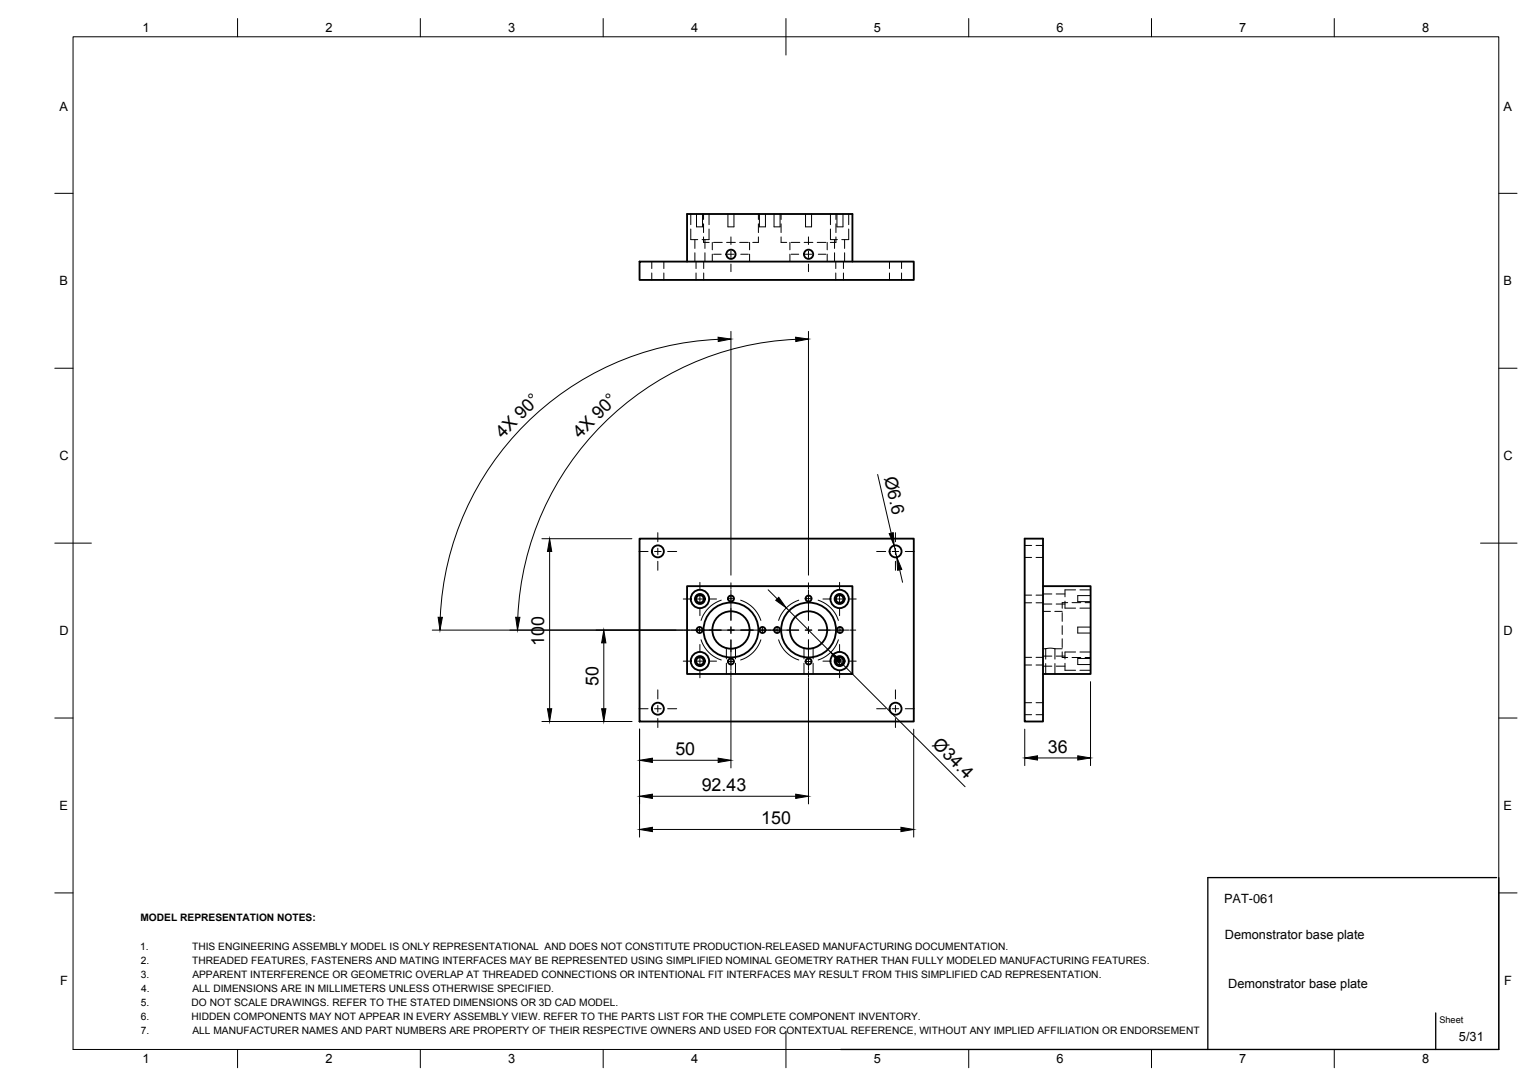
ISO-10303-21;
HEADER;
/* Generated by software containing ST-Developer
 * from STEP Tools, Inc. (www.steptools.com) 
 */

FILE_DESCRIPTION(
/* description */ ('Compact intermittent indexer'),
/* implementation_level */ '2;1');

FILE_NAME(
/* name */ 'Demonstrator base plate.step',
/* time_stamp */ '2026-10-29T16:32:17-07:00',
/* author */ (''),
/* organization */ (''),
/* preprocessor_version */ 'ST-DEVELOPER v20.2',
/* originating_system */ 'Autodesk Translation Framework v15.17.0.0',
/* authorisation */ '');

FILE_SCHEMA (('AUTOMOTIVE_DESIGN { 1 0 10303 214 3 1 1 }'));
ENDSEC;

DATA;
#10=MECHANICAL_DESIGN_GEOMETRIC_PRESENTATION_REPRESENTATION('',(#257),#10837);
#209=SHAPE_REPRESENTATION_RELATIONSHIP('SRR','None',#10943,#233);
#233=ADVANCED_BREP_SHAPE_REPRESENTATION('',(#289),#10810);
#257=STYLED_ITEM('',(#11145),#289);
#289=MANIFOLD_SOLID_BREP('Body1',#5629);
#319=B_SPLINE_CURVE_WITH_KNOTS('',3,(#8545,#8546,#8547,#8548,#8549,#8550,
#8551,#8552,#8553,#8554,#8555,#8556,#8557,#8558,#8559,#8560,#8561,#8562,
#8563,#8564,#8565,#8566,#8567,#8568,#8569,#8570,#8571,#8572,#8573,#8574,
#8575,#8576,#8577,#8578),.UNSPECIFIED.,.T.,.F.,(4,2,2,2,2,2,2,2,2,2,2,2,
2,2,2,2,4),(0.,0.094594182476448,0.189188364952896,0.283770357603024,0.378352350253152,
0.472934342903279,0.567516335553407,0.662110518029855,0.756704700506303,
0.851298882982751,0.945893065459199,1.04047505810933,1.13505705075945,1.22963904340958,
1.32422103605971,1.41881521853616,1.51340940101261),.UNSPECIFIED.);
#320=B_SPLINE_CURVE_WITH_KNOTS('',3,(#8621,#8622,#8623,#8624,#8625,#8626,
#8627,#8628,#8629,#8630,#8631,#8632,#8633,#8634,#8635,#8636,#8637,#8638,
#8639,#8640,#8641,#8642,#8643,#8644,#8645,#8646,#8647,#8648,#8649,#8650,
#8651,#8652,#8653,#8654),.UNSPECIFIED.,.T.,.F.,(4,2,2,2,2,2,2,2,2,2,2,2,
2,2,2,2,4),(0.,0.0945941824764479,0.189188364952896,0.283770357603024,0.378352350253152,
0.47293434290328,0.567516335553408,0.662110518029856,0.756704700506303,
0.851298882982751,0.945893065459199,1.04047505810933,1.13505705075946,1.22963904340958,
1.32422103605971,1.41881521853616,1.51340940101261),.UNSPECIFIED.);
#359=FACE_BOUND('',#996,.T.);
#360=FACE_BOUND('',#998,.T.);
#361=FACE_BOUND('',#1009,.T.);
#362=FACE_BOUND('',#1011,.T.);
#363=FACE_BOUND('',#1014,.T.);
#364=FACE_BOUND('',#1017,.T.);
#365=FACE_BOUND('',#1020,.T.);
#366=FACE_BOUND('',#1023,.T.);
#367=FACE_BOUND('',#1029,.T.);
#368=FACE_BOUND('',#1031,.T.);
#369=FACE_BOUND('',#1033,.T.);
#370=FACE_BOUND('',#1035,.T.);
#371=FACE_BOUND('',#1044,.T.);
#372=FACE_BOUND('',#1045,.T.);
#373=FACE_BOUND('',#1046,.T.);
#374=FACE_BOUND('',#1047,.T.);
#375=FACE_BOUND('',#1048,.T.);
#376=FACE_BOUND('',#1049,.T.);
#377=FACE_BOUND('',#1050,.T.);
#378=FACE_BOUND('',#1051,.T.);
#379=FACE_BOUND('',#1052,.T.);
#380=FACE_BOUND('',#1053,.T.);
#381=FACE_BOUND('',#1054,.T.);
#382=FACE_BOUND('',#1055,.T.);
#383=FACE_BOUND('',#1056,.T.);
#384=FACE_BOUND('',#1057,.T.);
#385=FACE_BOUND('',#1059,.T.);
#386=FACE_BOUND('',#1060,.T.);
#387=FACE_BOUND('',#1074,.T.);
#388=FACE_BOUND('',#1075,.T.);
#389=FACE_BOUND('',#1076,.T.);
#390=FACE_BOUND('',#1077,.T.);
#391=FACE_BOUND('',#1078,.T.);
#392=FACE_BOUND('',#1080,.T.);
#393=FACE_BOUND('',#1081,.T.);
#394=FACE_BOUND('',#1082,.T.);
#395=FACE_BOUND('',#1083,.T.);
#396=FACE_BOUND('',#1084,.T.);
#397=FACE_BOUND('',#1085,.T.);
#398=FACE_BOUND('',#1086,.T.);
#399=FACE_BOUND('',#1087,.T.);
#471=PLANE('',#5934);
#472=PLANE('',#5938);
#473=PLANE('',#5942);
#474=PLANE('',#5946);
#475=PLANE('',#5950);
#476=PLANE('',#5957);
#477=PLANE('',#5961);
#478=PLANE('',#5965);
#479=PLANE('',#5969);
#480=PLANE('',#5973);
#481=PLANE('',#5980);
#482=PLANE('',#5985);
#483=PLANE('',#5990);
#484=PLANE('',#5995);
#485=PLANE('',#6005);
#486=PLANE('',#6007);
#487=PLANE('',#6009);
#488=PLANE('',#6011);
#489=PLANE('',#6013);
#490=PLANE('',#6014);
#491=PLANE('',#6015);
#492=PLANE('',#6016);
#493=PLANE('',#6017);
#494=PLANE('',#6022);
#495=PLANE('',#6023);
#496=PLANE('',#6036);
#497=PLANE('',#6037);
#498=PLANE('',#6038);
#499=PLANE('',#6039);
#500=PLANE('',#6048);
#501=PLANE('',#6049);
#652=FACE_OUTER_BOUND('',#986,.T.);
#653=FACE_OUTER_BOUND('',#987,.T.);
#654=FACE_OUTER_BOUND('',#988,.T.);
#655=FACE_OUTER_BOUND('',#989,.T.);
#656=FACE_OUTER_BOUND('',#990,.T.);
#657=FACE_OUTER_BOUND('',#991,.T.);
#658=FACE_OUTER_BOUND('',#992,.T.);
#659=FACE_OUTER_BOUND('',#993,.T.);
#660=FACE_OUTER_BOUND('',#994,.T.);
#661=FACE_OUTER_BOUND('',#995,.T.);
#662=FACE_OUTER_BOUND('',#997,.T.);
#663=FACE_OUTER_BOUND('',#999,.T.);
#664=FACE_OUTER_BOUND('',#1000,.T.);
#665=FACE_OUTER_BOUND('',#1001,.T.);
#666=FACE_OUTER_BOUND('',#1002,.T.);
#667=FACE_OUTER_BOUND('',#1003,.T.);
#668=FACE_OUTER_BOUND('',#1004,.T.);
#669=FACE_OUTER_BOUND('',#1005,.T.);
#670=FACE_OUTER_BOUND('',#1006,.T.);
#671=FACE_OUTER_BOUND('',#1007,.T.);
#672=FACE_OUTER_BOUND('',#1008,.T.);
#673=FACE_OUTER_BOUND('',#1010,.T.);
#674=FACE_OUTER_BOUND('',#1012,.T.);
#675=FACE_OUTER_BOUND('',#1013,.T.);
#676=FACE_OUTER_BOUND('',#1015,.T.);
#677=FACE_OUTER_BOUND('',#1016,.T.);
#678=FACE_OUTER_BOUND('',#1018,.T.);
#679=FACE_OUTER_BOUND('',#1019,.T.);
#680=FACE_OUTER_BOUND('',#1021,.T.);
#681=FACE_OUTER_BOUND('',#1022,.T.);
#682=FACE_OUTER_BOUND('',#1024,.T.);
#683=FACE_OUTER_BOUND('',#1025,.T.);
#684=FACE_OUTER_BOUND('',#1026,.T.);
#685=FACE_OUTER_BOUND('',#1027,.T.);
#686=FACE_OUTER_BOUND('',#1028,.T.);
#687=FACE_OUTER_BOUND('',#1030,.T.);
#688=FACE_OUTER_BOUND('',#1032,.T.);
#689=FACE_OUTER_BOUND('',#1034,.T.);
#690=FACE_OUTER_BOUND('',#1036,.T.);
#691=FACE_OUTER_BOUND('',#1037,.T.);
#692=FACE_OUTER_BOUND('',#1038,.T.);
#693=FACE_OUTER_BOUND('',#1039,.T.);
#694=FACE_OUTER_BOUND('',#1040,.T.);
#695=FACE_OUTER_BOUND('',#1041,.T.);
#696=FACE_OUTER_BOUND('',#1042,.T.);
#697=FACE_OUTER_BOUND('',#1043,.T.);
#698=FACE_OUTER_BOUND('',#1058,.T.);
#699=FACE_OUTER_BOUND('',#1061,.T.);
#700=FACE_OUTER_BOUND('',#1062,.T.);
#701=FACE_OUTER_BOUND('',#1063,.T.);
#702=FACE_OUTER_BOUND('',#1064,.T.);
#703=FACE_OUTER_BOUND('',#1065,.T.);
#704=FACE_OUTER_BOUND('',#1066,.T.);
#705=FACE_OUTER_BOUND('',#1067,.T.);
#706=FACE_OUTER_BOUND('',#1068,.T.);
#707=FACE_OUTER_BOUND('',#1069,.T.);
#708=FACE_OUTER_BOUND('',#1070,.T.);
#709=FACE_OUTER_BOUND('',#1071,.T.);
#710=FACE_OUTER_BOUND('',#1072,.T.);
#711=FACE_OUTER_BOUND('',#1073,.T.);
#712=FACE_OUTER_BOUND('',#1079,.T.);
#986=EDGE_LOOP('',(#3708,#3709,#3710,#3711));
#987=EDGE_LOOP('',(#3712));
#988=EDGE_LOOP('',(#3713,#3714,#3715,#3716));
#989=EDGE_LOOP('',(#3717));
#990=EDGE_LOOP('',(#3718,#3719,#3720,#3721));
#991=EDGE_LOOP('',(#3722));
#992=EDGE_LOOP('',(#3723,#3724,#3725,#3726));
#993=EDGE_LOOP('',(#3727));
#994=EDGE_LOOP('',(#3728,#3729,#3730,#3731));
#995=EDGE_LOOP('',(#3732));
#996=EDGE_LOOP('',(#3733));
#997=EDGE_LOOP('',(#3734,#3735,#3736,#3737));
#998=EDGE_LOOP('',(#3738));
#999=EDGE_LOOP('',(#3739,#3740,#3741,#3742));
#1000=EDGE_LOOP('',(#3743));
#1001=EDGE_LOOP('',(#3744,#3745,#3746,#3747));
#1002=EDGE_LOOP('',(#3748));
#1003=EDGE_LOOP('',(#3749,#3750,#3751,#3752));
#1004=EDGE_LOOP('',(#3753));
#1005=EDGE_LOOP('',(#3754,#3755,#3756,#3757));
#1006=EDGE_LOOP('',(#3758));
#1007=EDGE_LOOP('',(#3759,#3760,#3761,#3762));
#1008=EDGE_LOOP('',(#3763));
#1009=EDGE_LOOP('',(#3764));
#1010=EDGE_LOOP('',(#3765,#3766,#3767,#3768));
#1011=EDGE_LOOP('',(#3769));
#1012=EDGE_LOOP('',(#3770,#3771,#3772,#3773));
#1013=EDGE_LOOP('',(#3774));
#1014=EDGE_LOOP('',(#3775));
#1015=EDGE_LOOP('',(#3776,#3777,#3778,#3779));
#1016=EDGE_LOOP('',(#3780));
#1017=EDGE_LOOP('',(#3781));
#1018=EDGE_LOOP('',(#3782,#3783,#3784,#3785));
#1019=EDGE_LOOP('',(#3786));
#1020=EDGE_LOOP('',(#3787));
#1021=EDGE_LOOP('',(#3788,#3789,#3790,#3791));
#1022=EDGE_LOOP('',(#3792));
#1023=EDGE_LOOP('',(#3793));
#1024=EDGE_LOOP('',(#3794,#3795,#3796,#3797));
#1025=EDGE_LOOP('',(#3798,#3799,#3800,#3801));
#1026=EDGE_LOOP('',(#3802,#3803,#3804,#3805));
#1027=EDGE_LOOP('',(#3806,#3807,#3808,#3809));
#1028=EDGE_LOOP('',(#3810));
#1029=EDGE_LOOP('',(#3811));
#1030=EDGE_LOOP('',(#3812));
#1031=EDGE_LOOP('',(#3813));
#1032=EDGE_LOOP('',(#3814));
#1033=EDGE_LOOP('',(#3815));
#1034=EDGE_LOOP('',(#3816));
#1035=EDGE_LOOP('',(#3817));
#1036=EDGE_LOOP('',(#3818));
#1037=EDGE_LOOP('',(#3819));
#1038=EDGE_LOOP('',(#3820,#3821,#3822,#3823));
#1039=EDGE_LOOP('',(#3824,#3825,#3826,#3827));
#1040=EDGE_LOOP('',(#3828,#3829,#3830,#3831));
#1041=EDGE_LOOP('',(#3832,#3833,#3834,#3835));
#1042=EDGE_LOOP('',(#3836,#3837,#3838,#3839));
#1043=EDGE_LOOP('',(#3840,#3841,#3842,#3843));
#1044=EDGE_LOOP('',(#3844));
#1045=EDGE_LOOP('',(#3845));
#1046=EDGE_LOOP('',(#3846));
#1047=EDGE_LOOP('',(#3847));
#1048=EDGE_LOOP('',(#3848));
#1049=EDGE_LOOP('',(#3849));
#1050=EDGE_LOOP('',(#3850));
#1051=EDGE_LOOP('',(#3851));
#1052=EDGE_LOOP('',(#3852));
#1053=EDGE_LOOP('',(#3853));
#1054=EDGE_LOOP('',(#3854));
#1055=EDGE_LOOP('',(#3855));
#1056=EDGE_LOOP('',(#3856));
#1057=EDGE_LOOP('',(#3857));
#1058=EDGE_LOOP('',(#3858,#3859,#3860,#3861));
#1059=EDGE_LOOP('',(#3862));
#1060=EDGE_LOOP('',(#3863));
#1061=EDGE_LOOP('',(#3864,#3865,#3866,#3867));
#1062=EDGE_LOOP('',(#3868,#3869,#3870,#3871));
#1063=EDGE_LOOP('',(#3872,#3873,#3874,#3875));
#1064=EDGE_LOOP('',(#3876,#3877,#3878,#3879));
#1065=EDGE_LOOP('',(#3880,#3881,#3882,#3883));
#1066=EDGE_LOOP('',(#3884,#3885,#3886,#3887));
#1067=EDGE_LOOP('',(#3888,#3889,#3890,#3891));
#1068=EDGE_LOOP('',(#3892,#3893,#3894,#3895));
#1069=EDGE_LOOP('',(#3896,#3897,#3898,#3899));
#1070=EDGE_LOOP('',(#3900,#3901,#3902,#3903));
#1071=EDGE_LOOP('',(#3904,#3905,#3906,#3907));
#1072=EDGE_LOOP('',(#3908,#3909,#3910,#3911));
#1073=EDGE_LOOP('',(#3912,#3913,#3914,#3915));
#1074=EDGE_LOOP('',(#3916,#3917,#3918,#3919));
#1075=EDGE_LOOP('',(#3920));
#1076=EDGE_LOOP('',(#3921));
#1077=EDGE_LOOP('',(#3922));
#1078=EDGE_LOOP('',(#3923));
#1079=EDGE_LOOP('',(#3924,#3925,#3926,#3927));
#1080=EDGE_LOOP('',(#3928));
#1081=EDGE_LOOP('',(#3929));
#1082=EDGE_LOOP('',(#3930));
#1083=EDGE_LOOP('',(#3931));
#1084=EDGE_LOOP('',(#3932));
#1085=EDGE_LOOP('',(#3933));
#1086=EDGE_LOOP('',(#3934));
#1087=EDGE_LOOP('',(#3935));
#1432=LINE('',#8507,#1790);
#1433=LINE('',#8514,#1791);
#1434=LINE('',#8521,#1792);
#1435=LINE('',#8528,#1793);
#1436=LINE('',#8535,#1794);
#1437=LINE('',#8543,#1795);
#1438=LINE('',#8583,#1796);
#1439=LINE('',#8590,#1797);
#1440=LINE('',#8597,#1798);
#1441=LINE('',#8604,#1799);
#1442=LINE('',#8611,#1800);
#1443=LINE('',#8619,#1801);
#1444=LINE('',#8659,#1802);
#1445=LINE('',#8668,#1803);
#1446=LINE('',#8677,#1804);
#1447=LINE('',#8686,#1805);
#1448=LINE('',#8694,#1806);
#1449=LINE('',#8698,#1807);
#1450=LINE('',#8702,#1808);
#1451=LINE('',#8706,#1809);
#1452=LINE('',#8724,#1810);
#1453=LINE('',#8726,#1811);
#1454=LINE('',#8728,#1812);
#1455=LINE('',#8729,#1813);
#1456=LINE('',#8732,#1814);
#1457=LINE('',#8734,#1815);
#1458=LINE('',#8735,#1816);
#1459=LINE('',#8738,#1817);
#1460=LINE('',#8740,#1818);
#1461=LINE('',#8741,#1819);
#1462=LINE('',#8745,#1820);
#1463=LINE('',#8749,#1821);
#1464=LINE('',#8751,#1822);
#1465=LINE('',#8753,#1823);
#1466=LINE('',#8758,#1824);
#1467=LINE('',#8764,#1825);
#1468=LINE('',#8770,#1826);
#1469=LINE('',#8776,#1827);
#1470=LINE('',#8781,#1828);
#1471=LINE('',#8783,#1829);
#1472=LINE('',#8785,#1830);
#1473=LINE('',#8786,#1831);
#1474=LINE('',#8789,#1832);
#1475=LINE('',#8791,#1833);
#1476=LINE('',#8792,#1834);
#1477=LINE('',#8795,#1835);
#1478=LINE('',#8797,#1836);
#1479=LINE('',#8798,#1837);
#1480=LINE('',#8800,#1838);
#1481=LINE('',#8801,#1839);
#1482=LINE('',#8805,#1840);
#1483=LINE('',#8809,#1841);
#1484=LINE('',#8813,#1842);
#1485=LINE('',#8817,#1843);
#1790=VECTOR('',#6676,0.165);
#1791=VECTOR('',#6685,0.165);
#1792=VECTOR('',#6694,0.165);
#1793=VECTOR('',#6703,0.165);
#1794=VECTOR('',#6712,1.5);
#1795=VECTOR('',#6723,1.02);
#1796=VECTOR('',#6728,0.165);
#1797=VECTOR('',#6737,0.165);
#1798=VECTOR('',#6746,0.165);
#1799=VECTOR('',#6755,0.165);
#1800=VECTOR('',#6764,1.5);
#1801=VECTOR('',#6775,1.02);
#1802=VECTOR('',#6780,0.5);
#1803=VECTOR('',#6791,0.5);
#1804=VECTOR('',#6802,0.5);
#1805=VECTOR('',#6813,0.5);
#1806=VECTOR('',#6824,0.275);
#1807=VECTOR('',#6829,0.275);
#1808=VECTOR('',#6834,0.275);
#1809=VECTOR('',#6839,0.275);
#1810=VECTOR('',#6862,1.);
#1811=VECTOR('',#6863,1.);
#1812=VECTOR('',#6864,1.);
#1813=VECTOR('',#6865,1.);
#1814=VECTOR('',#6868,1.);
#1815=VECTOR('',#6869,1.);
#1816=VECTOR('',#6870,1.);
#1817=VECTOR('',#6873,1.);
#1818=VECTOR('',#6874,1.);
#1819=VECTOR('',#6875,1.);
#1820=VECTOR('',#6880,0.25);
#1821=VECTOR('',#6885,0.25);
#1822=VECTOR('',#6888,1.);
#1823=VECTOR('',#6891,1.);
#1824=VECTOR('',#6896,0.33);
#1825=VECTOR('',#6903,0.33);
#1826=VECTOR('',#6910,0.33);
#1827=VECTOR('',#6917,0.33);
#1828=VECTOR('',#6922,1.);
#1829=VECTOR('',#6923,1.);
#1830=VECTOR('',#6924,1.);
#1831=VECTOR('',#6925,1.);
#1832=VECTOR('',#6928,1.);
#1833=VECTOR('',#6929,1.);
#1834=VECTOR('',#6930,1.);
#1835=VECTOR('',#6933,1.);
#1836=VECTOR('',#6934,1.);
#1837=VECTOR('',#6935,1.);
#1838=VECTOR('',#6938,1.);
#1839=VECTOR('',#6939,1.);
#1840=VECTOR('',#6944,0.21);
#1841=VECTOR('',#6949,0.21);
#1842=VECTOR('',#6954,0.21);
#1843=VECTOR('',#6959,0.21);
#2148=CIRCLE('',#5932,0.165);
#2149=CIRCLE('',#5933,0.165);
#2150=CIRCLE('',#5936,0.165);
#2151=CIRCLE('',#5937,0.165);
#2152=CIRCLE('',#5940,0.165);
#2153=CIRCLE('',#5941,0.165);
#2154=CIRCLE('',#5944,0.165);
#2155=CIRCLE('',#5945,0.165);
#2156=CIRCLE('',#5948,1.5);
#2157=CIRCLE('',#5949,1.5);
#2158=CIRCLE('',#5951,1.02);
#2159=CIRCLE('',#5953,1.02);
#2160=CIRCLE('',#5955,0.165);
#2161=CIRCLE('',#5956,0.165);
#2162=CIRCLE('',#5959,0.165);
#2163=CIRCLE('',#5960,0.165);
#2164=CIRCLE('',#5963,0.165);
#2165=CIRCLE('',#5964,0.165);
#2166=CIRCLE('',#5967,0.165);
#2167=CIRCLE('',#5968,0.165);
#2168=CIRCLE('',#5971,1.5);
#2169=CIRCLE('',#5972,1.5);
#2170=CIRCLE('',#5974,1.02);
#2171=CIRCLE('',#5976,1.02);
#2172=CIRCLE('',#5978,0.5);
#2173=CIRCLE('',#5979,0.5);
#2174=CIRCLE('',#5981,0.275);
#2175=CIRCLE('',#5983,0.5);
#2176=CIRCLE('',#5984,0.5);
#2177=CIRCLE('',#5986,0.275);
#2178=CIRCLE('',#5988,0.5);
#2179=CIRCLE('',#5989,0.5);
#2180=CIRCLE('',#5991,0.275);
#2181=CIRCLE('',#5993,0.5);
#2182=CIRCLE('',#5994,0.5);
#2183=CIRCLE('',#5996,0.275);
#2184=CIRCLE('',#5998,0.275);
#2185=CIRCLE('',#6000,0.275);
#2186=CIRCLE('',#6002,0.275);
#2187=CIRCLE('',#6004,0.275);
#2188=CIRCLE('',#6006,0.21);
#2189=CIRCLE('',#6008,0.21);
#2190=CIRCLE('',#6010,0.21);
#2191=CIRCLE('',#6012,0.21);
#2192=CIRCLE('',#6019,0.25);
#2193=CIRCLE('',#6021,0.25);
#2194=CIRCLE('',#6025,0.33);
#2195=CIRCLE('',#6026,0.33);
#2196=CIRCLE('',#6028,0.33);
#2197=CIRCLE('',#6029,0.33);
#2198=CIRCLE('',#6031,0.33);
#2199=CIRCLE('',#6032,0.33);
#2200=CIRCLE('',#6034,0.33);
#2201=CIRCLE('',#6035,0.33);
#2202=CIRCLE('',#6041,0.21);
#2203=CIRCLE('',#6043,0.21);
#2204=CIRCLE('',#6045,0.21);
#2205=CIRCLE('',#6047,0.21);
#2482=VERTEX_POINT('',#8504);
#2483=VERTEX_POINT('',#8506);
#2484=VERTEX_POINT('',#8511);
#2485=VERTEX_POINT('',#8513);
#2486=VERTEX_POINT('',#8518);
#2487=VERTEX_POINT('',#8520);
#2488=VERTEX_POINT('',#8525);
#2489=VERTEX_POINT('',#8527);
#2490=VERTEX_POINT('',#8532);
#2491=VERTEX_POINT('',#8534);
#2492=VERTEX_POINT('',#8538);
#2493=VERTEX_POINT('',#8541);
#2494=VERTEX_POINT('',#8544);
#2495=VERTEX_POINT('',#8580);
#2496=VERTEX_POINT('',#8582);
#2497=VERTEX_POINT('',#8587);
#2498=VERTEX_POINT('',#8589);
#2499=VERTEX_POINT('',#8594);
#2500=VERTEX_POINT('',#8596);
#2501=VERTEX_POINT('',#8601);
#2502=VERTEX_POINT('',#8603);
#2503=VERTEX_POINT('',#8608);
#2504=VERTEX_POINT('',#8610);
#2505=VERTEX_POINT('',#8614);
#2506=VERTEX_POINT('',#8617);
#2507=VERTEX_POINT('',#8620);
#2508=VERTEX_POINT('',#8656);
#2509=VERTEX_POINT('',#8658);
#2510=VERTEX_POINT('',#8662);
#2511=VERTEX_POINT('',#8665);
#2512=VERTEX_POINT('',#8667);
#2513=VERTEX_POINT('',#8671);
#2514=VERTEX_POINT('',#8674);
#2515=VERTEX_POINT('',#8676);
#2516=VERTEX_POINT('',#8680);
#2517=VERTEX_POINT('',#8683);
#2518=VERTEX_POINT('',#8685);
#2519=VERTEX_POINT('',#8689);
#2520=VERTEX_POINT('',#8692);
#2521=VERTEX_POINT('',#8696);
#2522=VERTEX_POINT('',#8700);
#2523=VERTEX_POINT('',#8704);
#2524=VERTEX_POINT('',#8708);
#2525=VERTEX_POINT('',#8711);
#2526=VERTEX_POINT('',#8714);
#2527=VERTEX_POINT('',#8717);
#2528=VERTEX_POINT('',#8722);
#2529=VERTEX_POINT('',#8723);
#2530=VERTEX_POINT('',#8725);
#2531=VERTEX_POINT('',#8727);
#2532=VERTEX_POINT('',#8731);
#2533=VERTEX_POINT('',#8733);
#2534=VERTEX_POINT('',#8737);
#2535=VERTEX_POINT('',#8739);
#2536=VERTEX_POINT('',#8743);
#2537=VERTEX_POINT('',#8747);
#2538=VERTEX_POINT('',#8755);
#2539=VERTEX_POINT('',#8757);
#2540=VERTEX_POINT('',#8761);
#2541=VERTEX_POINT('',#8763);
#2542=VERTEX_POINT('',#8767);
#2543=VERTEX_POINT('',#8769);
#2544=VERTEX_POINT('',#8773);
#2545=VERTEX_POINT('',#8775);
#2546=VERTEX_POINT('',#8779);
#2547=VERTEX_POINT('',#8780);
#2548=VERTEX_POINT('',#8782);
#2549=VERTEX_POINT('',#8784);
#2550=VERTEX_POINT('',#8788);
#2551=VERTEX_POINT('',#8790);
#2552=VERTEX_POINT('',#8794);
#2553=VERTEX_POINT('',#8796);
#2554=VERTEX_POINT('',#8803);
#2555=VERTEX_POINT('',#8807);
#2556=VERTEX_POINT('',#8811);
#2557=VERTEX_POINT('',#8815);
#2976=EDGE_CURVE('',#2482,#2482,#2148,.T.);
#2977=EDGE_CURVE('',#2482,#2483,#1432,.T.);
#2978=EDGE_CURVE('',#2483,#2483,#2149,.T.);
#2979=EDGE_CURVE('',#2484,#2484,#2150,.T.);
#2980=EDGE_CURVE('',#2484,#2485,#1433,.T.);
#2981=EDGE_CURVE('',#2485,#2485,#2151,.T.);
#2982=EDGE_CURVE('',#2486,#2486,#2152,.T.);
#2983=EDGE_CURVE('',#2486,#2487,#1434,.T.);
#2984=EDGE_CURVE('',#2487,#2487,#2153,.T.);
#2985=EDGE_CURVE('',#2488,#2488,#2154,.T.);
#2986=EDGE_CURVE('',#2488,#2489,#1435,.T.);
#2987=EDGE_CURVE('',#2489,#2489,#2155,.T.);
#2988=EDGE_CURVE('',#2490,#2490,#2156,.T.);
#2989=EDGE_CURVE('',#2490,#2491,#1436,.T.);
#2990=EDGE_CURVE('',#2491,#2491,#2157,.T.);
#2991=EDGE_CURVE('',#2492,#2492,#2158,.T.);
#2992=EDGE_CURVE('',#2493,#2493,#2159,.T.);
#2993=EDGE_CURVE('',#2493,#2492,#1437,.T.);
#2994=EDGE_CURVE('',#2494,#2494,#319,.T.);
#2995=EDGE_CURVE('',#2495,#2495,#2160,.T.);
#2996=EDGE_CURVE('',#2495,#2496,#1438,.T.);
#2997=EDGE_CURVE('',#2496,#2496,#2161,.T.);
#2998=EDGE_CURVE('',#2497,#2497,#2162,.T.);
#2999=EDGE_CURVE('',#2497,#2498,#1439,.T.);
#3000=EDGE_CURVE('',#2498,#2498,#2163,.T.);
#3001=EDGE_CURVE('',#2499,#2499,#2164,.T.);
#3002=EDGE_CURVE('',#2499,#2500,#1440,.T.);
#3003=EDGE_CURVE('',#2500,#2500,#2165,.T.);
#3004=EDGE_CURVE('',#2501,#2501,#2166,.T.);
#3005=EDGE_CURVE('',#2501,#2502,#1441,.T.);
#3006=EDGE_CURVE('',#2502,#2502,#2167,.T.);
#3007=EDGE_CURVE('',#2503,#2503,#2168,.T.);
#3008=EDGE_CURVE('',#2503,#2504,#1442,.T.);
#3009=EDGE_CURVE('',#2504,#2504,#2169,.T.);
#3010=EDGE_CURVE('',#2505,#2505,#2170,.T.);
#3011=EDGE_CURVE('',#2506,#2506,#2171,.T.);
#3012=EDGE_CURVE('',#2506,#2505,#1443,.T.);
#3013=EDGE_CURVE('',#2507,#2507,#320,.T.);
#3014=EDGE_CURVE('',#2508,#2508,#2172,.T.);
#3015=EDGE_CURVE('',#2508,#2509,#1444,.T.);
#3016=EDGE_CURVE('',#2509,#2509,#2173,.T.);
#3017=EDGE_CURVE('',#2510,#2510,#2174,.T.);
#3018=EDGE_CURVE('',#2511,#2511,#2175,.T.);
#3019=EDGE_CURVE('',#2511,#2512,#1445,.T.);
#3020=EDGE_CURVE('',#2512,#2512,#2176,.T.);
#3021=EDGE_CURVE('',#2513,#2513,#2177,.T.);
#3022=EDGE_CURVE('',#2514,#2514,#2178,.T.);
#3023=EDGE_CURVE('',#2514,#2515,#1446,.T.);
#3024=EDGE_CURVE('',#2515,#2515,#2179,.T.);
#3025=EDGE_CURVE('',#2516,#2516,#2180,.T.);
#3026=EDGE_CURVE('',#2517,#2517,#2181,.T.);
#3027=EDGE_CURVE('',#2517,#2518,#1447,.T.);
#3028=EDGE_CURVE('',#2518,#2518,#2182,.T.);
#3029=EDGE_CURVE('',#2519,#2519,#2183,.T.);
#3030=EDGE_CURVE('',#2520,#2520,#2184,.T.);
#3031=EDGE_CURVE('',#2520,#2510,#1448,.T.);
#3032=EDGE_CURVE('',#2521,#2521,#2185,.T.);
#3033=EDGE_CURVE('',#2521,#2513,#1449,.T.);
#3034=EDGE_CURVE('',#2522,#2522,#2186,.T.);
#3035=EDGE_CURVE('',#2522,#2516,#1450,.T.);
#3036=EDGE_CURVE('',#2523,#2523,#2187,.T.);
#3037=EDGE_CURVE('',#2523,#2519,#1451,.T.);
#3038=EDGE_CURVE('',#2524,#2524,#2188,.T.);
#3039=EDGE_CURVE('',#2525,#2525,#2189,.T.);
#3040=EDGE_CURVE('',#2526,#2526,#2190,.T.);
#3041=EDGE_CURVE('',#2527,#2527,#2191,.T.);
#3042=EDGE_CURVE('',#2528,#2529,#1452,.T.);
#3043=EDGE_CURVE('',#2529,#2530,#1453,.T.);
#3044=EDGE_CURVE('',#2531,#2530,#1454,.T.);
#3045=EDGE_CURVE('',#2531,#2528,#1455,.T.);
#3046=EDGE_CURVE('',#2530,#2532,#1456,.T.);
#3047=EDGE_CURVE('',#2533,#2529,#1457,.T.);
#3048=EDGE_CURVE('',#2533,#2532,#1458,.T.);
#3049=EDGE_CURVE('',#2532,#2534,#1459,.T.);
#3050=EDGE_CURVE('',#2535,#2533,#1460,.T.);
#3051=EDGE_CURVE('',#2535,#2534,#1461,.T.);
#3052=EDGE_CURVE('',#2536,#2536,#2192,.T.);
#3053=EDGE_CURVE('',#2536,#2494,#1462,.T.);
#3054=EDGE_CURVE('',#2537,#2537,#2193,.T.);
#3055=EDGE_CURVE('',#2537,#2507,#1463,.T.);
#3056=EDGE_CURVE('',#2528,#2535,#1464,.T.);
#3057=EDGE_CURVE('',#2534,#2531,#1465,.T.);
#3058=EDGE_CURVE('',#2538,#2538,#2194,.T.);
#3059=EDGE_CURVE('',#2538,#2539,#1466,.T.);
#3060=EDGE_CURVE('',#2539,#2539,#2195,.T.);
#3061=EDGE_CURVE('',#2540,#2540,#2196,.T.);
#3062=EDGE_CURVE('',#2540,#2541,#1467,.T.);
#3063=EDGE_CURVE('',#2541,#2541,#2197,.T.);
#3064=EDGE_CURVE('',#2542,#2542,#2198,.T.);
#3065=EDGE_CURVE('',#2542,#2543,#1468,.T.);
#3066=EDGE_CURVE('',#2543,#2543,#2199,.T.);
#3067=EDGE_CURVE('',#2544,#2544,#2200,.T.);
#3068=EDGE_CURVE('',#2544,#2545,#1469,.T.);
#3069=EDGE_CURVE('',#2545,#2545,#2201,.T.);
#3070=EDGE_CURVE('',#2546,#2547,#1470,.T.);
#3071=EDGE_CURVE('',#2547,#2548,#1471,.T.);
#3072=EDGE_CURVE('',#2549,#2548,#1472,.T.);
#3073=EDGE_CURVE('',#2546,#2549,#1473,.T.);
#3074=EDGE_CURVE('',#2550,#2546,#1474,.T.);
#3075=EDGE_CURVE('',#2551,#2549,#1475,.T.);
#3076=EDGE_CURVE('',#2550,#2551,#1476,.T.);
#3077=EDGE_CURVE('',#2552,#2550,#1477,.T.);
#3078=EDGE_CURVE('',#2553,#2551,#1478,.T.);
#3079=EDGE_CURVE('',#2552,#2553,#1479,.T.);
#3080=EDGE_CURVE('',#2547,#2552,#1480,.T.);
#3081=EDGE_CURVE('',#2548,#2553,#1481,.T.);
#3082=EDGE_CURVE('',#2554,#2554,#2202,.T.);
#3083=EDGE_CURVE('',#2554,#2527,#1482,.T.);
#3084=EDGE_CURVE('',#2555,#2555,#2203,.T.);
#3085=EDGE_CURVE('',#2555,#2526,#1483,.T.);
#3086=EDGE_CURVE('',#2556,#2556,#2204,.T.);
#3087=EDGE_CURVE('',#2556,#2525,#1484,.T.);
#3088=EDGE_CURVE('',#2557,#2557,#2205,.T.);
#3089=EDGE_CURVE('',#2557,#2524,#1485,.T.);
#3708=ORIENTED_EDGE('',*,*,#2976,.F.);
#3709=ORIENTED_EDGE('',*,*,#2977,.T.);
#3710=ORIENTED_EDGE('',*,*,#2978,.F.);
#3711=ORIENTED_EDGE('',*,*,#2977,.F.);
#3712=ORIENTED_EDGE('',*,*,#2976,.T.);
#3713=ORIENTED_EDGE('',*,*,#2979,.F.);
#3714=ORIENTED_EDGE('',*,*,#2980,.T.);
#3715=ORIENTED_EDGE('',*,*,#2981,.F.);
#3716=ORIENTED_EDGE('',*,*,#2980,.F.);
#3717=ORIENTED_EDGE('',*,*,#2979,.T.);
#3718=ORIENTED_EDGE('',*,*,#2982,.F.);
#3719=ORIENTED_EDGE('',*,*,#2983,.T.);
#3720=ORIENTED_EDGE('',*,*,#2984,.F.);
#3721=ORIENTED_EDGE('',*,*,#2983,.F.);
#3722=ORIENTED_EDGE('',*,*,#2982,.T.);
#3723=ORIENTED_EDGE('',*,*,#2985,.F.);
#3724=ORIENTED_EDGE('',*,*,#2986,.T.);
#3725=ORIENTED_EDGE('',*,*,#2987,.F.);
#3726=ORIENTED_EDGE('',*,*,#2986,.F.);
#3727=ORIENTED_EDGE('',*,*,#2985,.T.);
#3728=ORIENTED_EDGE('',*,*,#2988,.F.);
#3729=ORIENTED_EDGE('',*,*,#2989,.T.);
#3730=ORIENTED_EDGE('',*,*,#2990,.F.);
#3731=ORIENTED_EDGE('',*,*,#2989,.F.);
#3732=ORIENTED_EDGE('',*,*,#2988,.T.);
#3733=ORIENTED_EDGE('',*,*,#2991,.F.);
#3734=ORIENTED_EDGE('',*,*,#2992,.F.);
#3735=ORIENTED_EDGE('',*,*,#2993,.T.);
#3736=ORIENTED_EDGE('',*,*,#2991,.T.);
#3737=ORIENTED_EDGE('',*,*,#2993,.F.);
#3738=ORIENTED_EDGE('',*,*,#2994,.T.);
#3739=ORIENTED_EDGE('',*,*,#2995,.F.);
#3740=ORIENTED_EDGE('',*,*,#2996,.T.);
#3741=ORIENTED_EDGE('',*,*,#2997,.F.);
#3742=ORIENTED_EDGE('',*,*,#2996,.F.);
#3743=ORIENTED_EDGE('',*,*,#2995,.T.);
#3744=ORIENTED_EDGE('',*,*,#2998,.F.);
#3745=ORIENTED_EDGE('',*,*,#2999,.T.);
#3746=ORIENTED_EDGE('',*,*,#3000,.F.);
#3747=ORIENTED_EDGE('',*,*,#2999,.F.);
#3748=ORIENTED_EDGE('',*,*,#2998,.T.);
#3749=ORIENTED_EDGE('',*,*,#3001,.F.);
#3750=ORIENTED_EDGE('',*,*,#3002,.T.);
#3751=ORIENTED_EDGE('',*,*,#3003,.F.);
#3752=ORIENTED_EDGE('',*,*,#3002,.F.);
#3753=ORIENTED_EDGE('',*,*,#3001,.T.);
#3754=ORIENTED_EDGE('',*,*,#3004,.F.);
#3755=ORIENTED_EDGE('',*,*,#3005,.T.);
#3756=ORIENTED_EDGE('',*,*,#3006,.F.);
#3757=ORIENTED_EDGE('',*,*,#3005,.F.);
#3758=ORIENTED_EDGE('',*,*,#3004,.T.);
#3759=ORIENTED_EDGE('',*,*,#3007,.F.);
#3760=ORIENTED_EDGE('',*,*,#3008,.T.);
#3761=ORIENTED_EDGE('',*,*,#3009,.F.);
#3762=ORIENTED_EDGE('',*,*,#3008,.F.);
#3763=ORIENTED_EDGE('',*,*,#3007,.T.);
#3764=ORIENTED_EDGE('',*,*,#3010,.F.);
#3765=ORIENTED_EDGE('',*,*,#3011,.F.);
#3766=ORIENTED_EDGE('',*,*,#3012,.T.);
#3767=ORIENTED_EDGE('',*,*,#3010,.T.);
#3768=ORIENTED_EDGE('',*,*,#3012,.F.);
#3769=ORIENTED_EDGE('',*,*,#3013,.T.);
#3770=ORIENTED_EDGE('',*,*,#3014,.F.);
#3771=ORIENTED_EDGE('',*,*,#3015,.T.);
#3772=ORIENTED_EDGE('',*,*,#3016,.F.);
#3773=ORIENTED_EDGE('',*,*,#3015,.F.);
#3774=ORIENTED_EDGE('',*,*,#3014,.T.);
#3775=ORIENTED_EDGE('',*,*,#3017,.F.);
#3776=ORIENTED_EDGE('',*,*,#3018,.F.);
#3777=ORIENTED_EDGE('',*,*,#3019,.T.);
#3778=ORIENTED_EDGE('',*,*,#3020,.F.);
#3779=ORIENTED_EDGE('',*,*,#3019,.F.);
#3780=ORIENTED_EDGE('',*,*,#3018,.T.);
#3781=ORIENTED_EDGE('',*,*,#3021,.F.);
#3782=ORIENTED_EDGE('',*,*,#3022,.F.);
#3783=ORIENTED_EDGE('',*,*,#3023,.T.);
#3784=ORIENTED_EDGE('',*,*,#3024,.F.);
#3785=ORIENTED_EDGE('',*,*,#3023,.F.);
#3786=ORIENTED_EDGE('',*,*,#3022,.T.);
#3787=ORIENTED_EDGE('',*,*,#3025,.F.);
#3788=ORIENTED_EDGE('',*,*,#3026,.F.);
#3789=ORIENTED_EDGE('',*,*,#3027,.T.);
#3790=ORIENTED_EDGE('',*,*,#3028,.F.);
#3791=ORIENTED_EDGE('',*,*,#3027,.F.);
#3792=ORIENTED_EDGE('',*,*,#3026,.T.);
#3793=ORIENTED_EDGE('',*,*,#3029,.F.);
#3794=ORIENTED_EDGE('',*,*,#3030,.F.);
#3795=ORIENTED_EDGE('',*,*,#3031,.T.);
#3796=ORIENTED_EDGE('',*,*,#3017,.T.);
#3797=ORIENTED_EDGE('',*,*,#3031,.F.);
#3798=ORIENTED_EDGE('',*,*,#3032,.F.);
#3799=ORIENTED_EDGE('',*,*,#3033,.T.);
#3800=ORIENTED_EDGE('',*,*,#3021,.T.);
#3801=ORIENTED_EDGE('',*,*,#3033,.F.);
#3802=ORIENTED_EDGE('',*,*,#3034,.F.);
#3803=ORIENTED_EDGE('',*,*,#3035,.T.);
#3804=ORIENTED_EDGE('',*,*,#3025,.T.);
#3805=ORIENTED_EDGE('',*,*,#3035,.F.);
#3806=ORIENTED_EDGE('',*,*,#3036,.F.);
#3807=ORIENTED_EDGE('',*,*,#3037,.T.);
#3808=ORIENTED_EDGE('',*,*,#3029,.T.);
#3809=ORIENTED_EDGE('',*,*,#3037,.F.);
#3810=ORIENTED_EDGE('',*,*,#3036,.T.);
#3811=ORIENTED_EDGE('',*,*,#3038,.T.);
#3812=ORIENTED_EDGE('',*,*,#3034,.T.);
#3813=ORIENTED_EDGE('',*,*,#3039,.T.);
#3814=ORIENTED_EDGE('',*,*,#3032,.T.);
#3815=ORIENTED_EDGE('',*,*,#3040,.T.);
#3816=ORIENTED_EDGE('',*,*,#3030,.T.);
#3817=ORIENTED_EDGE('',*,*,#3041,.T.);
#3818=ORIENTED_EDGE('',*,*,#3011,.T.);
#3819=ORIENTED_EDGE('',*,*,#2992,.T.);
#3820=ORIENTED_EDGE('',*,*,#3042,.T.);
#3821=ORIENTED_EDGE('',*,*,#3043,.T.);
#3822=ORIENTED_EDGE('',*,*,#3044,.F.);
#3823=ORIENTED_EDGE('',*,*,#3045,.T.);
#3824=ORIENTED_EDGE('',*,*,#3046,.F.);
#3825=ORIENTED_EDGE('',*,*,#3043,.F.);
#3826=ORIENTED_EDGE('',*,*,#3047,.F.);
#3827=ORIENTED_EDGE('',*,*,#3048,.T.);
#3828=ORIENTED_EDGE('',*,*,#3049,.F.);
#3829=ORIENTED_EDGE('',*,*,#3048,.F.);
#3830=ORIENTED_EDGE('',*,*,#3050,.F.);
#3831=ORIENTED_EDGE('',*,*,#3051,.T.);
#3832=ORIENTED_EDGE('',*,*,#3052,.F.);
#3833=ORIENTED_EDGE('',*,*,#3053,.T.);
#3834=ORIENTED_EDGE('',*,*,#2994,.F.);
#3835=ORIENTED_EDGE('',*,*,#3053,.F.);
#3836=ORIENTED_EDGE('',*,*,#3054,.F.);
#3837=ORIENTED_EDGE('',*,*,#3055,.T.);
#3838=ORIENTED_EDGE('',*,*,#3013,.F.);
#3839=ORIENTED_EDGE('',*,*,#3055,.F.);
#3840=ORIENTED_EDGE('',*,*,#3056,.T.);
#3841=ORIENTED_EDGE('',*,*,#3050,.T.);
#3842=ORIENTED_EDGE('',*,*,#3047,.T.);
#3843=ORIENTED_EDGE('',*,*,#3042,.F.);
#3844=ORIENTED_EDGE('',*,*,#3020,.T.);
#3845=ORIENTED_EDGE('',*,*,#3024,.T.);
#3846=ORIENTED_EDGE('',*,*,#3028,.T.);
#3847=ORIENTED_EDGE('',*,*,#2978,.T.);
#3848=ORIENTED_EDGE('',*,*,#2981,.T.);
#3849=ORIENTED_EDGE('',*,*,#2984,.T.);
#3850=ORIENTED_EDGE('',*,*,#2987,.T.);
#3851=ORIENTED_EDGE('',*,*,#2990,.T.);
#3852=ORIENTED_EDGE('',*,*,#3009,.T.);
#3853=ORIENTED_EDGE('',*,*,#3006,.T.);
#3854=ORIENTED_EDGE('',*,*,#3003,.T.);
#3855=ORIENTED_EDGE('',*,*,#3000,.T.);
#3856=ORIENTED_EDGE('',*,*,#2997,.T.);
#3857=ORIENTED_EDGE('',*,*,#3016,.T.);
#3858=ORIENTED_EDGE('',*,*,#3057,.F.);
#3859=ORIENTED_EDGE('',*,*,#3051,.F.);
#3860=ORIENTED_EDGE('',*,*,#3056,.F.);
#3861=ORIENTED_EDGE('',*,*,#3045,.F.);
#3862=ORIENTED_EDGE('',*,*,#3054,.T.);
#3863=ORIENTED_EDGE('',*,*,#3052,.T.);
#3864=ORIENTED_EDGE('',*,*,#3058,.F.);
#3865=ORIENTED_EDGE('',*,*,#3059,.T.);
#3866=ORIENTED_EDGE('',*,*,#3060,.F.);
#3867=ORIENTED_EDGE('',*,*,#3059,.F.);
#3868=ORIENTED_EDGE('',*,*,#3061,.F.);
#3869=ORIENTED_EDGE('',*,*,#3062,.T.);
#3870=ORIENTED_EDGE('',*,*,#3063,.F.);
#3871=ORIENTED_EDGE('',*,*,#3062,.F.);
#3872=ORIENTED_EDGE('',*,*,#3064,.F.);
#3873=ORIENTED_EDGE('',*,*,#3065,.T.);
#3874=ORIENTED_EDGE('',*,*,#3066,.F.);
#3875=ORIENTED_EDGE('',*,*,#3065,.F.);
#3876=ORIENTED_EDGE('',*,*,#3067,.F.);
#3877=ORIENTED_EDGE('',*,*,#3068,.T.);
#3878=ORIENTED_EDGE('',*,*,#3069,.F.);
#3879=ORIENTED_EDGE('',*,*,#3068,.F.);
#3880=ORIENTED_EDGE('',*,*,#3070,.T.);
#3881=ORIENTED_EDGE('',*,*,#3071,.T.);
#3882=ORIENTED_EDGE('',*,*,#3072,.F.);
#3883=ORIENTED_EDGE('',*,*,#3073,.F.);
#3884=ORIENTED_EDGE('',*,*,#3074,.T.);
#3885=ORIENTED_EDGE('',*,*,#3073,.T.);
#3886=ORIENTED_EDGE('',*,*,#3075,.F.);
#3887=ORIENTED_EDGE('',*,*,#3076,.F.);
#3888=ORIENTED_EDGE('',*,*,#3077,.T.);
#3889=ORIENTED_EDGE('',*,*,#3076,.T.);
#3890=ORIENTED_EDGE('',*,*,#3078,.F.);
#3891=ORIENTED_EDGE('',*,*,#3079,.F.);
#3892=ORIENTED_EDGE('',*,*,#3080,.T.);
#3893=ORIENTED_EDGE('',*,*,#3079,.T.);
#3894=ORIENTED_EDGE('',*,*,#3081,.F.);
#3895=ORIENTED_EDGE('',*,*,#3071,.F.);
#3896=ORIENTED_EDGE('',*,*,#3082,.F.);
#3897=ORIENTED_EDGE('',*,*,#3083,.T.);
#3898=ORIENTED_EDGE('',*,*,#3041,.F.);
#3899=ORIENTED_EDGE('',*,*,#3083,.F.);
#3900=ORIENTED_EDGE('',*,*,#3084,.F.);
#3901=ORIENTED_EDGE('',*,*,#3085,.T.);
#3902=ORIENTED_EDGE('',*,*,#3040,.F.);
#3903=ORIENTED_EDGE('',*,*,#3085,.F.);
#3904=ORIENTED_EDGE('',*,*,#3086,.F.);
#3905=ORIENTED_EDGE('',*,*,#3087,.T.);
#3906=ORIENTED_EDGE('',*,*,#3039,.F.);
#3907=ORIENTED_EDGE('',*,*,#3087,.F.);
#3908=ORIENTED_EDGE('',*,*,#3088,.F.);
#3909=ORIENTED_EDGE('',*,*,#3089,.T.);
#3910=ORIENTED_EDGE('',*,*,#3038,.F.);
#3911=ORIENTED_EDGE('',*,*,#3089,.F.);
#3912=ORIENTED_EDGE('',*,*,#3078,.T.);
#3913=ORIENTED_EDGE('',*,*,#3075,.T.);
#3914=ORIENTED_EDGE('',*,*,#3072,.T.);
#3915=ORIENTED_EDGE('',*,*,#3081,.T.);
#3916=ORIENTED_EDGE('',*,*,#3057,.T.);
#3917=ORIENTED_EDGE('',*,*,#3044,.T.);
#3918=ORIENTED_EDGE('',*,*,#3046,.T.);
#3919=ORIENTED_EDGE('',*,*,#3049,.T.);
#3920=ORIENTED_EDGE('',*,*,#3069,.T.);
#3921=ORIENTED_EDGE('',*,*,#3066,.T.);
#3922=ORIENTED_EDGE('',*,*,#3063,.T.);
#3923=ORIENTED_EDGE('',*,*,#3060,.T.);
#3924=ORIENTED_EDGE('',*,*,#3070,.F.);
#3925=ORIENTED_EDGE('',*,*,#3074,.F.);
#3926=ORIENTED_EDGE('',*,*,#3077,.F.);
#3927=ORIENTED_EDGE('',*,*,#3080,.F.);
#3928=ORIENTED_EDGE('',*,*,#3088,.T.);
#3929=ORIENTED_EDGE('',*,*,#3086,.T.);
#3930=ORIENTED_EDGE('',*,*,#3084,.T.);
#3931=ORIENTED_EDGE('',*,*,#3082,.T.);
#3932=ORIENTED_EDGE('',*,*,#3067,.T.);
#3933=ORIENTED_EDGE('',*,*,#3064,.T.);
#3934=ORIENTED_EDGE('',*,*,#3061,.T.);
#3935=ORIENTED_EDGE('',*,*,#3058,.T.);
#5172=CYLINDRICAL_SURFACE('',#5931,0.165);
#5173=CYLINDRICAL_SURFACE('',#5935,0.165);
#5174=CYLINDRICAL_SURFACE('',#5939,0.165);
#5175=CYLINDRICAL_SURFACE('',#5943,0.165);
#5176=CYLINDRICAL_SURFACE('',#5947,1.5);
#5177=CYLINDRICAL_SURFACE('',#5952,1.02);
#5178=CYLINDRICAL_SURFACE('',#5954,0.165);
#5179=CYLINDRICAL_SURFACE('',#5958,0.165);
#5180=CYLINDRICAL_SURFACE('',#5962,0.165);
#5181=CYLINDRICAL_SURFACE('',#5966,0.165);
#5182=CYLINDRICAL_SURFACE('',#5970,1.5);
#5183=CYLINDRICAL_SURFACE('',#5975,1.02);
#5184=CYLINDRICAL_SURFACE('',#5977,0.5);
#5185=CYLINDRICAL_SURFACE('',#5982,0.5);
#5186=CYLINDRICAL_SURFACE('',#5987,0.5);
#5187=CYLINDRICAL_SURFACE('',#5992,0.5);
#5188=CYLINDRICAL_SURFACE('',#5997,0.275);
#5189=CYLINDRICAL_SURFACE('',#5999,0.275);
#5190=CYLINDRICAL_SURFACE('',#6001,0.275);
#5191=CYLINDRICAL_SURFACE('',#6003,0.275);
#5192=CYLINDRICAL_SURFACE('',#6018,0.25);
#5193=CYLINDRICAL_SURFACE('',#6020,0.25);
#5194=CYLINDRICAL_SURFACE('',#6024,0.33);
#5195=CYLINDRICAL_SURFACE('',#6027,0.33);
#5196=CYLINDRICAL_SURFACE('',#6030,0.33);
#5197=CYLINDRICAL_SURFACE('',#6033,0.33);
#5198=CYLINDRICAL_SURFACE('',#6040,0.21);
#5199=CYLINDRICAL_SURFACE('',#6042,0.21);
#5200=CYLINDRICAL_SURFACE('',#6044,0.21);
#5201=CYLINDRICAL_SURFACE('',#6046,0.21);
#5295=ADVANCED_FACE('',(#652),#5172,.F.);
#5296=ADVANCED_FACE('',(#653),#471,.T.);
#5297=ADVANCED_FACE('',(#654),#5173,.F.);
#5298=ADVANCED_FACE('',(#655),#472,.T.);
#5299=ADVANCED_FACE('',(#656),#5174,.F.);
#5300=ADVANCED_FACE('',(#657),#473,.T.);
#5301=ADVANCED_FACE('',(#658),#5175,.F.);
#5302=ADVANCED_FACE('',(#659),#474,.T.);
#5303=ADVANCED_FACE('',(#660),#5176,.F.);
#5304=ADVANCED_FACE('',(#661,#359),#475,.T.);
#5305=ADVANCED_FACE('',(#662,#360),#5177,.F.);
#5306=ADVANCED_FACE('',(#663),#5178,.F.);
#5307=ADVANCED_FACE('',(#664),#476,.T.);
#5308=ADVANCED_FACE('',(#665),#5179,.F.);
#5309=ADVANCED_FACE('',(#666),#477,.T.);
#5310=ADVANCED_FACE('',(#667),#5180,.F.);
#5311=ADVANCED_FACE('',(#668),#478,.T.);
#5312=ADVANCED_FACE('',(#669),#5181,.F.);
#5313=ADVANCED_FACE('',(#670),#479,.T.);
#5314=ADVANCED_FACE('',(#671),#5182,.F.);
#5315=ADVANCED_FACE('',(#672,#361),#480,.T.);
#5316=ADVANCED_FACE('',(#673,#362),#5183,.F.);
#5317=ADVANCED_FACE('',(#674),#5184,.F.);
#5318=ADVANCED_FACE('',(#675,#363),#481,.T.);
#5319=ADVANCED_FACE('',(#676),#5185,.F.);
#5320=ADVANCED_FACE('',(#677,#364),#482,.T.);
#5321=ADVANCED_FACE('',(#678),#5186,.F.);
#5322=ADVANCED_FACE('',(#679,#365),#483,.T.);
#5323=ADVANCED_FACE('',(#680),#5187,.F.);
#5324=ADVANCED_FACE('',(#681,#366),#484,.T.);
#5325=ADVANCED_FACE('',(#682),#5188,.F.);
#5326=ADVANCED_FACE('',(#683),#5189,.F.);
#5327=ADVANCED_FACE('',(#684),#5190,.F.);
#5328=ADVANCED_FACE('',(#685),#5191,.F.);
#5329=ADVANCED_FACE('',(#686,#367),#485,.T.);
#5330=ADVANCED_FACE('',(#687,#368),#486,.T.);
#5331=ADVANCED_FACE('',(#688,#369),#487,.T.);
#5332=ADVANCED_FACE('',(#689,#370),#488,.T.);
#5333=ADVANCED_FACE('',(#690),#489,.T.);
#5334=ADVANCED_FACE('',(#691),#490,.T.);
#5335=ADVANCED_FACE('',(#692),#491,.T.);
#5336=ADVANCED_FACE('',(#693),#492,.T.);
#5337=ADVANCED_FACE('',(#694),#493,.T.);
#5338=ADVANCED_FACE('',(#695),#5192,.F.);
#5339=ADVANCED_FACE('',(#696),#5193,.F.);
#5340=ADVANCED_FACE('',(#697,#371,#372,#373,#374,#375,#376,#377,#378,#379,
#380,#381,#382,#383,#384),#494,.T.);
#5341=ADVANCED_FACE('',(#698,#385,#386),#495,.T.);
#5342=ADVANCED_FACE('',(#699),#5194,.F.);
#5343=ADVANCED_FACE('',(#700),#5195,.F.);
#5344=ADVANCED_FACE('',(#701),#5196,.F.);
#5345=ADVANCED_FACE('',(#702),#5197,.F.);
#5346=ADVANCED_FACE('',(#703),#496,.T.);
#5347=ADVANCED_FACE('',(#704),#497,.T.);
#5348=ADVANCED_FACE('',(#705),#498,.T.);
#5349=ADVANCED_FACE('',(#706),#499,.T.);
#5350=ADVANCED_FACE('',(#707),#5198,.F.);
#5351=ADVANCED_FACE('',(#708),#5199,.F.);
#5352=ADVANCED_FACE('',(#709),#5200,.F.);
#5353=ADVANCED_FACE('',(#710),#5201,.F.);
#5354=ADVANCED_FACE('',(#711,#387,#388,#389,#390,#391),#500,.T.);
#5355=ADVANCED_FACE('',(#712,#392,#393,#394,#395,#396,#397,#398,#399),#501,
 .F.);
#5629=CLOSED_SHELL('',(#5295,#5296,#5297,#5298,#5299,#5300,#5301,#5302,
#5303,#5304,#5305,#5306,#5307,#5308,#5309,#5310,#5311,#5312,#5313,#5314,
#5315,#5316,#5317,#5318,#5319,#5320,#5321,#5322,#5323,#5324,#5325,#5326,
#5327,#5328,#5329,#5330,#5331,#5332,#5333,#5334,#5335,#5336,#5337,#5338,
#5339,#5340,#5341,#5342,#5343,#5344,#5345,#5346,#5347,#5348,#5349,#5350,
#5351,#5352,#5353,#5354,#5355));
#5930=AXIS2_PLACEMENT_3D('',#8502,#6670,#6671);
#5931=AXIS2_PLACEMENT_3D('',#8503,#6672,#6673);
#5932=AXIS2_PLACEMENT_3D('',#8505,#6674,#6675);
#5933=AXIS2_PLACEMENT_3D('',#8508,#6677,#6678);
#5934=AXIS2_PLACEMENT_3D('',#8509,#6679,#6680);
#5935=AXIS2_PLACEMENT_3D('',#8510,#6681,#6682);
#5936=AXIS2_PLACEMENT_3D('',#8512,#6683,#6684);
#5937=AXIS2_PLACEMENT_3D('',#8515,#6686,#6687);
#5938=AXIS2_PLACEMENT_3D('',#8516,#6688,#6689);
#5939=AXIS2_PLACEMENT_3D('',#8517,#6690,#6691);
#5940=AXIS2_PLACEMENT_3D('',#8519,#6692,#6693);
#5941=AXIS2_PLACEMENT_3D('',#8522,#6695,#6696);
#5942=AXIS2_PLACEMENT_3D('',#8523,#6697,#6698);
#5943=AXIS2_PLACEMENT_3D('',#8524,#6699,#6700);
#5944=AXIS2_PLACEMENT_3D('',#8526,#6701,#6702);
#5945=AXIS2_PLACEMENT_3D('',#8529,#6704,#6705);
#5946=AXIS2_PLACEMENT_3D('',#8530,#6706,#6707);
#5947=AXIS2_PLACEMENT_3D('',#8531,#6708,#6709);
#5948=AXIS2_PLACEMENT_3D('',#8533,#6710,#6711);
#5949=AXIS2_PLACEMENT_3D('',#8536,#6713,#6714);
#5950=AXIS2_PLACEMENT_3D('',#8537,#6715,#6716);
#5951=AXIS2_PLACEMENT_3D('',#8539,#6717,#6718);
#5952=AXIS2_PLACEMENT_3D('',#8540,#6719,#6720);
#5953=AXIS2_PLACEMENT_3D('',#8542,#6721,#6722);
#5954=AXIS2_PLACEMENT_3D('',#8579,#6724,#6725);
#5955=AXIS2_PLACEMENT_3D('',#8581,#6726,#6727);
#5956=AXIS2_PLACEMENT_3D('',#8584,#6729,#6730);
#5957=AXIS2_PLACEMENT_3D('',#8585,#6731,#6732);
#5958=AXIS2_PLACEMENT_3D('',#8586,#6733,#6734);
#5959=AXIS2_PLACEMENT_3D('',#8588,#6735,#6736);
#5960=AXIS2_PLACEMENT_3D('',#8591,#6738,#6739);
#5961=AXIS2_PLACEMENT_3D('',#8592,#6740,#6741);
#5962=AXIS2_PLACEMENT_3D('',#8593,#6742,#6743);
#5963=AXIS2_PLACEMENT_3D('',#8595,#6744,#6745);
#5964=AXIS2_PLACEMENT_3D('',#8598,#6747,#6748);
#5965=AXIS2_PLACEMENT_3D('',#8599,#6749,#6750);
#5966=AXIS2_PLACEMENT_3D('',#8600,#6751,#6752);
#5967=AXIS2_PLACEMENT_3D('',#8602,#6753,#6754);
#5968=AXIS2_PLACEMENT_3D('',#8605,#6756,#6757);
#5969=AXIS2_PLACEMENT_3D('',#8606,#6758,#6759);
#5970=AXIS2_PLACEMENT_3D('',#8607,#6760,#6761);
#5971=AXIS2_PLACEMENT_3D('',#8609,#6762,#6763);
#5972=AXIS2_PLACEMENT_3D('',#8612,#6765,#6766);
#5973=AXIS2_PLACEMENT_3D('',#8613,#6767,#6768);
#5974=AXIS2_PLACEMENT_3D('',#8615,#6769,#6770);
#5975=AXIS2_PLACEMENT_3D('',#8616,#6771,#6772);
#5976=AXIS2_PLACEMENT_3D('',#8618,#6773,#6774);
#5977=AXIS2_PLACEMENT_3D('',#8655,#6776,#6777);
#5978=AXIS2_PLACEMENT_3D('',#8657,#6778,#6779);
#5979=AXIS2_PLACEMENT_3D('',#8660,#6781,#6782);
#5980=AXIS2_PLACEMENT_3D('',#8661,#6783,#6784);
#5981=AXIS2_PLACEMENT_3D('',#8663,#6785,#6786);
#5982=AXIS2_PLACEMENT_3D('',#8664,#6787,#6788);
#5983=AXIS2_PLACEMENT_3D('',#8666,#6789,#6790);
#5984=AXIS2_PLACEMENT_3D('',#8669,#6792,#6793);
#5985=AXIS2_PLACEMENT_3D('',#8670,#6794,#6795);
#5986=AXIS2_PLACEMENT_3D('',#8672,#6796,#6797);
#5987=AXIS2_PLACEMENT_3D('',#8673,#6798,#6799);
#5988=AXIS2_PLACEMENT_3D('',#8675,#6800,#6801);
#5989=AXIS2_PLACEMENT_3D('',#8678,#6803,#6804);
#5990=AXIS2_PLACEMENT_3D('',#8679,#6805,#6806);
#5991=AXIS2_PLACEMENT_3D('',#8681,#6807,#6808);
#5992=AXIS2_PLACEMENT_3D('',#8682,#6809,#6810);
#5993=AXIS2_PLACEMENT_3D('',#8684,#6811,#6812);
#5994=AXIS2_PLACEMENT_3D('',#8687,#6814,#6815);
#5995=AXIS2_PLACEMENT_3D('',#8688,#6816,#6817);
#5996=AXIS2_PLACEMENT_3D('',#8690,#6818,#6819);
#5997=AXIS2_PLACEMENT_3D('',#8691,#6820,#6821);
#5998=AXIS2_PLACEMENT_3D('',#8693,#6822,#6823);
#5999=AXIS2_PLACEMENT_3D('',#8695,#6825,#6826);
#6000=AXIS2_PLACEMENT_3D('',#8697,#6827,#6828);
#6001=AXIS2_PLACEMENT_3D('',#8699,#6830,#6831);
#6002=AXIS2_PLACEMENT_3D('',#8701,#6832,#6833);
#6003=AXIS2_PLACEMENT_3D('',#8703,#6835,#6836);
#6004=AXIS2_PLACEMENT_3D('',#8705,#6837,#6838);
#6005=AXIS2_PLACEMENT_3D('',#8707,#6840,#6841);
#6006=AXIS2_PLACEMENT_3D('',#8709,#6842,#6843);
#6007=AXIS2_PLACEMENT_3D('',#8710,#6844,#6845);
#6008=AXIS2_PLACEMENT_3D('',#8712,#6846,#6847);
#6009=AXIS2_PLACEMENT_3D('',#8713,#6848,#6849);
#6010=AXIS2_PLACEMENT_3D('',#8715,#6850,#6851);
#6011=AXIS2_PLACEMENT_3D('',#8716,#6852,#6853);
#6012=AXIS2_PLACEMENT_3D('',#8718,#6854,#6855);
#6013=AXIS2_PLACEMENT_3D('',#8719,#6856,#6857);
#6014=AXIS2_PLACEMENT_3D('',#8720,#6858,#6859);
#6015=AXIS2_PLACEMENT_3D('',#8721,#6860,#6861);
#6016=AXIS2_PLACEMENT_3D('',#8730,#6866,#6867);
#6017=AXIS2_PLACEMENT_3D('',#8736,#6871,#6872);
#6018=AXIS2_PLACEMENT_3D('',#8742,#6876,#6877);
#6019=AXIS2_PLACEMENT_3D('',#8744,#6878,#6879);
#6020=AXIS2_PLACEMENT_3D('',#8746,#6881,#6882);
#6021=AXIS2_PLACEMENT_3D('',#8748,#6883,#6884);
#6022=AXIS2_PLACEMENT_3D('',#8750,#6886,#6887);
#6023=AXIS2_PLACEMENT_3D('',#8752,#6889,#6890);
#6024=AXIS2_PLACEMENT_3D('',#8754,#6892,#6893);
#6025=AXIS2_PLACEMENT_3D('',#8756,#6894,#6895);
#6026=AXIS2_PLACEMENT_3D('',#8759,#6897,#6898);
#6027=AXIS2_PLACEMENT_3D('',#8760,#6899,#6900);
#6028=AXIS2_PLACEMENT_3D('',#8762,#6901,#6902);
#6029=AXIS2_PLACEMENT_3D('',#8765,#6904,#6905);
#6030=AXIS2_PLACEMENT_3D('',#8766,#6906,#6907);
#6031=AXIS2_PLACEMENT_3D('',#8768,#6908,#6909);
#6032=AXIS2_PLACEMENT_3D('',#8771,#6911,#6912);
#6033=AXIS2_PLACEMENT_3D('',#8772,#6913,#6914);
#6034=AXIS2_PLACEMENT_3D('',#8774,#6915,#6916);
#6035=AXIS2_PLACEMENT_3D('',#8777,#6918,#6919);
#6036=AXIS2_PLACEMENT_3D('',#8778,#6920,#6921);
#6037=AXIS2_PLACEMENT_3D('',#8787,#6926,#6927);
#6038=AXIS2_PLACEMENT_3D('',#8793,#6931,#6932);
#6039=AXIS2_PLACEMENT_3D('',#8799,#6936,#6937);
#6040=AXIS2_PLACEMENT_3D('',#8802,#6940,#6941);
#6041=AXIS2_PLACEMENT_3D('',#8804,#6942,#6943);
#6042=AXIS2_PLACEMENT_3D('',#8806,#6945,#6946);
#6043=AXIS2_PLACEMENT_3D('',#8808,#6947,#6948);
#6044=AXIS2_PLACEMENT_3D('',#8810,#6950,#6951);
#6045=AXIS2_PLACEMENT_3D('',#8812,#6952,#6953);
#6046=AXIS2_PLACEMENT_3D('',#8814,#6955,#6956);
#6047=AXIS2_PLACEMENT_3D('',#8816,#6957,#6958);
#6048=AXIS2_PLACEMENT_3D('',#8818,#6960,#6961);
#6049=AXIS2_PLACEMENT_3D('',#8819,#6962,#6963);
#6670=DIRECTION('axis',(0.,0.,1.));
#6671=DIRECTION('refdir',(1.,0.,0.));
#6672=DIRECTION('center_axis',(0.,0.,1.));
#6673=DIRECTION('ref_axis',(1.,0.,0.));
#6674=DIRECTION('center_axis',(0.,0.,1.));
#6675=DIRECTION('ref_axis',(1.,0.,0.));
#6676=DIRECTION('',(0.,0.,1.));
#6677=DIRECTION('center_axis',(0.,0.,-1.));
#6678=DIRECTION('ref_axis',(1.,0.,0.));
#6679=DIRECTION('center_axis',(0.,0.,1.));
#6680=DIRECTION('ref_axis',(1.,0.,0.));
#6681=DIRECTION('center_axis',(0.,0.,1.));
#6682=DIRECTION('ref_axis',(1.,0.,0.));
#6683=DIRECTION('center_axis',(0.,0.,1.));
#6684=DIRECTION('ref_axis',(1.,0.,0.));
#6685=DIRECTION('',(0.,0.,1.));
#6686=DIRECTION('center_axis',(0.,0.,-1.));
#6687=DIRECTION('ref_axis',(1.,0.,0.));
#6688=DIRECTION('center_axis',(0.,0.,1.));
#6689=DIRECTION('ref_axis',(1.,0.,0.));
#6690=DIRECTION('center_axis',(0.,0.,1.));
#6691=DIRECTION('ref_axis',(1.,0.,0.));
#6692=DIRECTION('center_axis',(0.,0.,1.));
#6693=DIRECTION('ref_axis',(1.,0.,0.));
#6694=DIRECTION('',(0.,0.,1.));
#6695=DIRECTION('center_axis',(0.,0.,-1.));
#6696=DIRECTION('ref_axis',(1.,0.,0.));
#6697=DIRECTION('center_axis',(0.,0.,1.));
#6698=DIRECTION('ref_axis',(1.,0.,0.));
#6699=DIRECTION('center_axis',(0.,0.,1.));
#6700=DIRECTION('ref_axis',(1.,0.,0.));
#6701=DIRECTION('center_axis',(0.,0.,1.));
#6702=DIRECTION('ref_axis',(1.,0.,0.));
#6703=DIRECTION('',(0.,0.,1.));
#6704=DIRECTION('center_axis',(0.,0.,-1.));
#6705=DIRECTION('ref_axis',(1.,0.,0.));
#6706=DIRECTION('center_axis',(0.,0.,1.));
#6707=DIRECTION('ref_axis',(1.,0.,0.));
#6708=DIRECTION('center_axis',(0.,0.,1.));
#6709=DIRECTION('ref_axis',(1.,0.,0.));
#6710=DIRECTION('center_axis',(0.,0.,1.));
#6711=DIRECTION('ref_axis',(1.,0.,0.));
#6712=DIRECTION('',(0.,0.,1.));
#6713=DIRECTION('center_axis',(0.,0.,-1.));
#6714=DIRECTION('ref_axis',(1.,0.,0.));
#6715=DIRECTION('center_axis',(0.,0.,1.));
#6716=DIRECTION('ref_axis',(1.,0.,0.));
#6717=DIRECTION('center_axis',(0.,0.,1.));
#6718=DIRECTION('ref_axis',(1.,0.,0.));
#6719=DIRECTION('center_axis',(0.,0.,1.));
#6720=DIRECTION('ref_axis',(1.,0.,0.));
#6721=DIRECTION('center_axis',(0.,0.,1.));
#6722=DIRECTION('ref_axis',(1.,0.,0.));
#6723=DIRECTION('',(0.,0.,1.));
#6724=DIRECTION('center_axis',(0.,0.,1.));
#6725=DIRECTION('ref_axis',(1.,0.,0.));
#6726=DIRECTION('center_axis',(0.,0.,1.));
#6727=DIRECTION('ref_axis',(1.,0.,0.));
#6728=DIRECTION('',(0.,0.,1.));
#6729=DIRECTION('center_axis',(0.,0.,-1.));
#6730=DIRECTION('ref_axis',(1.,0.,0.));
#6731=DIRECTION('center_axis',(0.,0.,1.));
#6732=DIRECTION('ref_axis',(1.,0.,0.));
#6733=DIRECTION('center_axis',(0.,0.,1.));
#6734=DIRECTION('ref_axis',(1.,0.,0.));
#6735=DIRECTION('center_axis',(0.,0.,1.));
#6736=DIRECTION('ref_axis',(1.,0.,0.));
#6737=DIRECTION('',(0.,0.,1.));
#6738=DIRECTION('center_axis',(0.,0.,-1.));
#6739=DIRECTION('ref_axis',(1.,0.,0.));
#6740=DIRECTION('center_axis',(0.,0.,1.));
#6741=DIRECTION('ref_axis',(1.,0.,0.));
#6742=DIRECTION('center_axis',(0.,0.,1.));
#6743=DIRECTION('ref_axis',(1.,0.,0.));
#6744=DIRECTION('center_axis',(0.,0.,1.));
#6745=DIRECTION('ref_axis',(1.,0.,0.));
#6746=DIRECTION('',(0.,0.,1.));
#6747=DIRECTION('center_axis',(0.,0.,-1.));
#6748=DIRECTION('ref_axis',(1.,0.,0.));
#6749=DIRECTION('center_axis',(0.,0.,1.));
#6750=DIRECTION('ref_axis',(1.,0.,0.));
#6751=DIRECTION('center_axis',(0.,0.,1.));
#6752=DIRECTION('ref_axis',(1.,0.,0.));
#6753=DIRECTION('center_axis',(0.,0.,1.));
#6754=DIRECTION('ref_axis',(1.,0.,0.));
#6755=DIRECTION('',(0.,0.,1.));
#6756=DIRECTION('center_axis',(0.,0.,-1.));
#6757=DIRECTION('ref_axis',(1.,0.,0.));
#6758=DIRECTION('center_axis',(0.,0.,1.));
#6759=DIRECTION('ref_axis',(1.,0.,0.));
#6760=DIRECTION('center_axis',(0.,0.,1.));
#6761=DIRECTION('ref_axis',(1.,0.,0.));
#6762=DIRECTION('center_axis',(0.,0.,1.));
#6763=DIRECTION('ref_axis',(1.,0.,0.));
#6764=DIRECTION('',(0.,0.,1.));
#6765=DIRECTION('center_axis',(0.,0.,-1.));
#6766=DIRECTION('ref_axis',(1.,0.,0.));
#6767=DIRECTION('center_axis',(0.,0.,1.));
#6768=DIRECTION('ref_axis',(1.,0.,0.));
#6769=DIRECTION('center_axis',(0.,0.,1.));
#6770=DIRECTION('ref_axis',(1.,0.,0.));
#6771=DIRECTION('center_axis',(0.,0.,1.));
#6772=DIRECTION('ref_axis',(1.,0.,0.));
#6773=DIRECTION('center_axis',(0.,0.,1.));
#6774=DIRECTION('ref_axis',(1.,0.,0.));
#6775=DIRECTION('',(0.,0.,1.));
#6776=DIRECTION('center_axis',(0.,0.,1.));
#6777=DIRECTION('ref_axis',(1.,0.,0.));
#6778=DIRECTION('center_axis',(0.,0.,1.));
#6779=DIRECTION('ref_axis',(1.,0.,0.));
#6780=DIRECTION('',(0.,0.,1.));
#6781=DIRECTION('center_axis',(0.,0.,-1.));
#6782=DIRECTION('ref_axis',(1.,0.,0.));
#6783=DIRECTION('center_axis',(0.,0.,1.));
#6784=DIRECTION('ref_axis',(1.,0.,0.));
#6785=DIRECTION('center_axis',(0.,0.,1.));
#6786=DIRECTION('ref_axis',(1.,0.,0.));
#6787=DIRECTION('center_axis',(0.,0.,1.));
#6788=DIRECTION('ref_axis',(1.,0.,0.));
#6789=DIRECTION('center_axis',(0.,0.,1.));
#6790=DIRECTION('ref_axis',(1.,0.,0.));
#6791=DIRECTION('',(0.,0.,1.));
#6792=DIRECTION('center_axis',(0.,0.,-1.));
#6793=DIRECTION('ref_axis',(1.,0.,0.));
#6794=DIRECTION('center_axis',(0.,0.,1.));
#6795=DIRECTION('ref_axis',(1.,0.,0.));
#6796=DIRECTION('center_axis',(0.,0.,1.));
#6797=DIRECTION('ref_axis',(1.,0.,0.));
#6798=DIRECTION('center_axis',(0.,0.,1.));
#6799=DIRECTION('ref_axis',(1.,0.,0.));
#6800=DIRECTION('center_axis',(0.,0.,1.));
#6801=DIRECTION('ref_axis',(1.,0.,0.));
#6802=DIRECTION('',(0.,0.,1.));
#6803=DIRECTION('center_axis',(0.,0.,-1.));
#6804=DIRECTION('ref_axis',(1.,0.,0.));
#6805=DIRECTION('center_axis',(0.,0.,1.));
#6806=DIRECTION('ref_axis',(1.,0.,0.));
#6807=DIRECTION('center_axis',(0.,0.,1.));
#6808=DIRECTION('ref_axis',(1.,0.,0.));
#6809=DIRECTION('center_axis',(0.,0.,1.));
#6810=DIRECTION('ref_axis',(1.,0.,0.));
#6811=DIRECTION('center_axis',(0.,0.,1.));
#6812=DIRECTION('ref_axis',(1.,0.,0.));
#6813=DIRECTION('',(0.,0.,1.));
#6814=DIRECTION('center_axis',(0.,0.,-1.));
#6815=DIRECTION('ref_axis',(1.,0.,0.));
#6816=DIRECTION('center_axis',(0.,0.,1.));
#6817=DIRECTION('ref_axis',(1.,0.,0.));
#6818=DIRECTION('center_axis',(0.,0.,1.));
#6819=DIRECTION('ref_axis',(1.,0.,0.));
#6820=DIRECTION('center_axis',(0.,0.,1.));
#6821=DIRECTION('ref_axis',(1.,0.,0.));
#6822=DIRECTION('center_axis',(0.,0.,1.));
#6823=DIRECTION('ref_axis',(1.,0.,0.));
#6824=DIRECTION('',(0.,0.,1.));
#6825=DIRECTION('center_axis',(0.,0.,1.));
#6826=DIRECTION('ref_axis',(1.,0.,0.));
#6827=DIRECTION('center_axis',(0.,0.,1.));
#6828=DIRECTION('ref_axis',(1.,0.,0.));
#6829=DIRECTION('',(0.,0.,1.));
#6830=DIRECTION('center_axis',(0.,0.,1.));
#6831=DIRECTION('ref_axis',(1.,0.,0.));
#6832=DIRECTION('center_axis',(0.,0.,1.));
#6833=DIRECTION('ref_axis',(1.,0.,0.));
#6834=DIRECTION('',(0.,0.,1.));
#6835=DIRECTION('center_axis',(0.,0.,1.));
#6836=DIRECTION('ref_axis',(1.,0.,0.));
#6837=DIRECTION('center_axis',(0.,0.,1.));
#6838=DIRECTION('ref_axis',(1.,0.,0.));
#6839=DIRECTION('',(0.,0.,1.));
#6840=DIRECTION('center_axis',(0.,0.,1.));
#6841=DIRECTION('ref_axis',(1.,0.,0.));
#6842=DIRECTION('center_axis',(0.,0.,-1.));
#6843=DIRECTION('ref_axis',(1.,0.,0.));
#6844=DIRECTION('center_axis',(0.,0.,1.));
#6845=DIRECTION('ref_axis',(1.,0.,0.));
#6846=DIRECTION('center_axis',(0.,0.,-1.));
#6847=DIRECTION('ref_axis',(1.,0.,0.));
#6848=DIRECTION('center_axis',(0.,0.,1.));
#6849=DIRECTION('ref_axis',(1.,0.,0.));
#6850=DIRECTION('center_axis',(0.,0.,-1.));
#6851=DIRECTION('ref_axis',(1.,0.,0.));
#6852=DIRECTION('center_axis',(0.,0.,1.));
#6853=DIRECTION('ref_axis',(1.,0.,0.));
#6854=DIRECTION('center_axis',(0.,0.,-1.));
#6855=DIRECTION('ref_axis',(1.,0.,0.));
#6856=DIRECTION('center_axis',(0.,0.,1.));
#6857=DIRECTION('ref_axis',(1.,0.,0.));
#6858=DIRECTION('center_axis',(0.,0.,1.));
#6859=DIRECTION('ref_axis',(1.,0.,0.));
#6860=DIRECTION('center_axis',(-1.,0.,0.));
#6861=DIRECTION('ref_axis',(0.,0.,1.));
#6862=DIRECTION('',(0.,1.,0.));
#6863=DIRECTION('',(0.,0.,-1.));
#6864=DIRECTION('',(0.,1.,0.));
#6865=DIRECTION('',(0.,0.,1.));
#6866=DIRECTION('center_axis',(0.,1.,0.));
#6867=DIRECTION('ref_axis',(0.,0.,1.));
#6868=DIRECTION('',(1.,0.,0.));
#6869=DIRECTION('',(-1.,0.,0.));
#6870=DIRECTION('',(0.,0.,-1.));
#6871=DIRECTION('center_axis',(1.,0.,0.));
#6872=DIRECTION('ref_axis',(0.,0.,-1.));
#6873=DIRECTION('',(0.,-1.,0.));
#6874=DIRECTION('',(0.,1.,0.));
#6875=DIRECTION('',(0.,0.,-1.));
#6876=DIRECTION('center_axis',(0.,-1.,0.));
#6877=DIRECTION('ref_axis',(1.,0.,0.));
#6878=DIRECTION('center_axis',(0.,1.,0.));
#6879=DIRECTION('ref_axis',(1.,0.,0.));
#6880=DIRECTION('',(0.,1.,0.));
#6881=DIRECTION('center_axis',(0.,-1.,0.));
#6882=DIRECTION('ref_axis',(1.,0.,0.));
#6883=DIRECTION('center_axis',(0.,1.,0.));
#6884=DIRECTION('ref_axis',(1.,0.,0.));
#6885=DIRECTION('',(0.,1.,0.));
#6886=DIRECTION('center_axis',(0.,0.,1.));
#6887=DIRECTION('ref_axis',(-1.,0.,0.));
#6888=DIRECTION('',(1.,0.,0.));
#6889=DIRECTION('center_axis',(0.,-1.,0.));
#6890=DIRECTION('ref_axis',(1.,0.,0.));
#6891=DIRECTION('',(-1.,0.,0.));
#6892=DIRECTION('center_axis',(0.,0.,1.));
#6893=DIRECTION('ref_axis',(1.,0.,0.));
#6894=DIRECTION('center_axis',(0.,0.,1.));
#6895=DIRECTION('ref_axis',(1.,0.,0.));
#6896=DIRECTION('',(0.,0.,1.));
#6897=DIRECTION('center_axis',(0.,0.,-1.));
#6898=DIRECTION('ref_axis',(1.,0.,0.));
#6899=DIRECTION('center_axis',(0.,0.,1.));
#6900=DIRECTION('ref_axis',(1.,0.,0.));
#6901=DIRECTION('center_axis',(0.,0.,1.));
#6902=DIRECTION('ref_axis',(1.,0.,0.));
#6903=DIRECTION('',(0.,0.,1.));
#6904=DIRECTION('center_axis',(0.,0.,-1.));
#6905=DIRECTION('ref_axis',(1.,0.,0.));
#6906=DIRECTION('center_axis',(0.,0.,1.));
#6907=DIRECTION('ref_axis',(1.,0.,0.));
#6908=DIRECTION('center_axis',(0.,0.,1.));
#6909=DIRECTION('ref_axis',(1.,0.,0.));
#6910=DIRECTION('',(0.,0.,1.));
#6911=DIRECTION('center_axis',(0.,0.,-1.));
#6912=DIRECTION('ref_axis',(1.,0.,0.));
#6913=DIRECTION('center_axis',(0.,0.,1.));
#6914=DIRECTION('ref_axis',(1.,0.,0.));
#6915=DIRECTION('center_axis',(0.,0.,1.));
#6916=DIRECTION('ref_axis',(1.,0.,0.));
#6917=DIRECTION('',(0.,0.,1.));
#6918=DIRECTION('center_axis',(0.,0.,-1.));
#6919=DIRECTION('ref_axis',(1.,0.,0.));
#6920=DIRECTION('center_axis',(0.,1.,0.));
#6921=DIRECTION('ref_axis',(-1.,0.,0.));
#6922=DIRECTION('',(-1.,0.,0.));
#6923=DIRECTION('',(0.,0.,1.));
#6924=DIRECTION('',(-1.,0.,0.));
#6925=DIRECTION('',(0.,0.,1.));
#6926=DIRECTION('center_axis',(1.,0.,0.));
#6927=DIRECTION('ref_axis',(0.,1.,0.));
#6928=DIRECTION('',(0.,1.,0.));
#6929=DIRECTION('',(0.,1.,0.));
#6930=DIRECTION('',(0.,0.,1.));
#6931=DIRECTION('center_axis',(0.,-1.,0.));
#6932=DIRECTION('ref_axis',(1.,0.,0.));
#6933=DIRECTION('',(1.,0.,0.));
#6934=DIRECTION('',(1.,0.,0.));
#6935=DIRECTION('',(0.,0.,1.));
#6936=DIRECTION('center_axis',(-1.,0.,0.));
#6937=DIRECTION('ref_axis',(0.,-1.,0.));
#6938=DIRECTION('',(0.,-1.,0.));
#6939=DIRECTION('',(0.,-1.,0.));
#6940=DIRECTION('center_axis',(0.,0.,1.));
#6941=DIRECTION('ref_axis',(1.,0.,0.));
#6942=DIRECTION('center_axis',(0.,0.,1.));
#6943=DIRECTION('ref_axis',(1.,0.,0.));
#6944=DIRECTION('',(0.,0.,1.));
#6945=DIRECTION('center_axis',(0.,0.,1.));
#6946=DIRECTION('ref_axis',(1.,0.,0.));
#6947=DIRECTION('center_axis',(0.,0.,1.));
#6948=DIRECTION('ref_axis',(1.,0.,0.));
#6949=DIRECTION('',(0.,0.,1.));
#6950=DIRECTION('center_axis',(0.,0.,1.));
#6951=DIRECTION('ref_axis',(1.,0.,0.));
#6952=DIRECTION('center_axis',(0.,0.,1.));
#6953=DIRECTION('ref_axis',(1.,0.,0.));
#6954=DIRECTION('',(0.,0.,1.));
#6955=DIRECTION('center_axis',(0.,0.,1.));
#6956=DIRECTION('ref_axis',(1.,0.,0.));
#6957=DIRECTION('center_axis',(0.,0.,1.));
#6958=DIRECTION('ref_axis',(1.,0.,0.));
#6959=DIRECTION('',(0.,0.,1.));
#6960=DIRECTION('center_axis',(0.,0.,1.));
#6961=DIRECTION('ref_axis',(1.,0.,0.));
#6962=DIRECTION('center_axis',(0.,0.,1.));
#6963=DIRECTION('ref_axis',(1.,0.,0.));
#8502=CARTESIAN_POINT('',(0.,0.,0.));
#8503=CARTESIAN_POINT('Origin',(2.52264068711929,2.10639249453345E-16,2.9));
#8504=CARTESIAN_POINT('',(2.35764068711929,1.90432577267413E-16,2.9));
#8505=CARTESIAN_POINT('Origin',(2.52264068711929,2.10639249453345E-16,2.9));
#8506=CARTESIAN_POINT('',(2.35764068711929,2.30845921639276E-16,3.6));
#8507=CARTESIAN_POINT('',(2.35764068711929,1.90432577267413E-16,2.9));
#8508=CARTESIAN_POINT('Origin',(2.52264068711929,2.10639249453345E-16,3.6));
#8509=CARTESIAN_POINT('Origin',(2.52264068711929,2.22044604925031E-16,2.9));
#8510=CARTESIAN_POINT('Origin',(4.24264068711929,1.72,2.9));
#8511=CARTESIAN_POINT('',(4.07764068711929,1.72,2.9));
#8512=CARTESIAN_POINT('Origin',(4.24264068711929,1.72,2.9));
#8513=CARTESIAN_POINT('',(4.07764068711929,1.72,3.6));
#8514=CARTESIAN_POINT('',(4.07764068711929,1.72,2.9));
#8515=CARTESIAN_POINT('Origin',(4.24264068711929,1.72,3.6));
#8516=CARTESIAN_POINT('Origin',(4.24264068711929,1.72,2.9));
#8517=CARTESIAN_POINT('Origin',(5.96264068711929,0.,2.9));
#8518=CARTESIAN_POINT('',(5.79764068711929,-2.02066721859313E-17,2.9));
#8519=CARTESIAN_POINT('Origin',(5.96264068711929,0.,2.9));
#8520=CARTESIAN_POINT('',(5.79764068711929,2.02066721859313E-17,3.6));
#8521=CARTESIAN_POINT('',(5.79764068711929,-2.02066721859313E-17,2.9));
#8522=CARTESIAN_POINT('Origin',(5.96264068711929,0.,3.6));
#8523=CARTESIAN_POINT('Origin',(5.96264068711929,0.,2.9));
#8524=CARTESIAN_POINT('Origin',(4.24264068711929,-1.72,2.9));
#8525=CARTESIAN_POINT('',(4.07764068711929,-1.72,2.9));
#8526=CARTESIAN_POINT('Origin',(4.24264068711929,-1.72,2.9));
#8527=CARTESIAN_POINT('',(4.07764068711929,-1.72,3.6));
#8528=CARTESIAN_POINT('',(4.07764068711929,-1.72,2.9));
#8529=CARTESIAN_POINT('Origin',(4.24264068711929,-1.72,3.6));
#8530=CARTESIAN_POINT('Origin',(4.24264068711929,-1.72,2.9));
#8531=CARTESIAN_POINT('Origin',(4.24264068711929,0.,2.05));
#8532=CARTESIAN_POINT('',(2.74264068711929,-1.83697019872103E-16,2.05));
#8533=CARTESIAN_POINT('Origin',(4.24264068711929,0.,2.05));
#8534=CARTESIAN_POINT('',(2.74264068711929,1.83697019872103E-16,3.6));
#8535=CARTESIAN_POINT('',(2.74264068711929,-1.83697019872103E-16,2.05));
#8536=CARTESIAN_POINT('Origin',(4.24264068711929,0.,3.6));
#8537=CARTESIAN_POINT('Origin',(4.24264068711929,0.,2.05));
#8538=CARTESIAN_POINT('',(3.22264068711929,-1.2491397351303E-16,2.05));
#8539=CARTESIAN_POINT('Origin',(4.24264068711929,0.,2.05));
#8540=CARTESIAN_POINT('Origin',(4.24264068711929,0.,0.9));
#8541=CARTESIAN_POINT('',(3.22264068711929,-1.2491397351303E-16,1.));
#8542=CARTESIAN_POINT('Origin',(4.24264068711929,0.,1.));
#8543=CARTESIAN_POINT('',(3.22264068711929,-1.2491397351303E-16,0.9));
#8544=CARTESIAN_POINT('',(3.99264068711929,-0.988888264668966,1.4));
#8545=CARTESIAN_POINT('Ctrl Pts',(3.99264068711929,-0.988888264668966,1.4));
#8546=CARTESIAN_POINT('Ctrl Pts',(3.99264068711929,-0.988888264668966,1.36846860584118));
#8547=CARTESIAN_POINT('Ctrl Pts',(3.99896863868788,-0.990553370646674,1.33492785033683));
#8548=CARTESIAN_POINT('Ctrl Pts',(4.02452085710491,-0.996491737296663,1.27337379025046));
#8549=CARTESIAN_POINT('Ctrl Pts',(4.04373855891321,-1.00067109353237,1.2453487376128));
#8550=CARTESIAN_POINT('Ctrl Pts',(4.08798657355057,-1.00845756932386,1.20110072297544));
#8551=CARTESIAN_POINT('Ctrl Pts',(4.11601281617403,-1.01258144235289,1.18188079690607));
#8552=CARTESIAN_POINT('Ctrl Pts',(4.17757108672792,-1.0183917429657,1.15632695599232));
#8553=CARTESIAN_POINT('Ctrl Pts',(4.21111335623591,-1.02,1.15));
#8554=CARTESIAN_POINT('Ctrl Pts',(4.27416801800266,-1.02,1.15));
#8555=CARTESIAN_POINT('Ctrl Pts',(4.30771028751065,-1.0183917429657,1.15632695599232));
#8556=CARTESIAN_POINT('Ctrl Pts',(4.36926855806454,-1.01258144235289,1.18188079690607));
#8557=CARTESIAN_POINT('Ctrl Pts',(4.397294800688,-1.00845756932386,1.20110072297544));
#8558=CARTESIAN_POINT('Ctrl Pts',(4.44154281532536,-1.00067109353237,1.2453487376128));
#8559=CARTESIAN_POINT('Ctrl Pts',(4.46076051713366,-0.996491737296663,1.27337379025046));
#8560=CARTESIAN_POINT('Ctrl Pts',(4.48631273555069,-0.990553370646674,1.33492785033683));
#8561=CARTESIAN_POINT('Ctrl Pts',(4.49264068711929,-0.988888264668966,1.36846860584118));
#8562=CARTESIAN_POINT('Ctrl Pts',(4.49264068711929,-0.988888264668966,1.43153139415882));
#8563=CARTESIAN_POINT('Ctrl Pts',(4.48631273555069,-0.990553370646674,1.46507214966317));
#8564=CARTESIAN_POINT('Ctrl Pts',(4.46076051713366,-0.996491737296663,1.52662620974954));
#8565=CARTESIAN_POINT('Ctrl Pts',(4.44154281532536,-1.00067109353237,1.5546512623872));
#8566=CARTESIAN_POINT('Ctrl Pts',(4.397294800688,-1.00845756932386,1.59889927702456));
#8567=CARTESIAN_POINT('Ctrl Pts',(4.36926855806454,-1.01258144235289,1.61811920309393));
#8568=CARTESIAN_POINT('Ctrl Pts',(4.30771028751065,-1.0183917429657,1.64367304400768));
#8569=CARTESIAN_POINT('Ctrl Pts',(4.27416801800266,-1.02,1.65));
#8570=CARTESIAN_POINT('Ctrl Pts',(4.21111335623591,-1.02,1.65));
#8571=CARTESIAN_POINT('Ctrl Pts',(4.17757108672792,-1.0183917429657,1.64367304400768));
#8572=CARTESIAN_POINT('Ctrl Pts',(4.11601281617403,-1.01258144235289,1.61811920309393));
#8573=CARTESIAN_POINT('Ctrl Pts',(4.08798657355057,-1.00845756932386,1.59889927702456));
#8574=CARTESIAN_POINT('Ctrl Pts',(4.04373855891321,-1.00067109353237,1.5546512623872));
#8575=CARTESIAN_POINT('Ctrl Pts',(4.02452085710491,-0.996491737296663,1.52662620974954));
#8576=CARTESIAN_POINT('Ctrl Pts',(3.99896863868788,-0.990553370646674,1.46507214966317));
#8577=CARTESIAN_POINT('Ctrl Pts',(3.99264068711929,-0.988888264668966,1.43153139415882));
#8578=CARTESIAN_POINT('Ctrl Pts',(3.99264068711929,-0.988888264668966,1.4));
#8579=CARTESIAN_POINT('Origin',(-1.72,2.10639249453345E-16,2.9));
#8580=CARTESIAN_POINT('',(-1.885,1.90432577267413E-16,2.9));
#8581=CARTESIAN_POINT('Origin',(-1.72,2.10639249453345E-16,2.9));
#8582=CARTESIAN_POINT('',(-1.885,2.30845921639276E-16,3.6));
#8583=CARTESIAN_POINT('',(-1.885,1.90432577267413E-16,2.9));
#8584=CARTESIAN_POINT('Origin',(-1.72,2.10639249453345E-16,3.6));
#8585=CARTESIAN_POINT('Origin',(-1.72,2.22044604925031E-16,2.9));
#8586=CARTESIAN_POINT('Origin',(1.05319624726672E-16,1.72,2.9));
#8587=CARTESIAN_POINT('',(-0.165,1.72,2.9));
#8588=CARTESIAN_POINT('Origin',(1.05319624726672E-16,1.72,2.9));
#8589=CARTESIAN_POINT('',(-0.165,1.72,3.6));
#8590=CARTESIAN_POINT('',(-0.165,1.72,2.9));
#8591=CARTESIAN_POINT('Origin',(1.05319624726672E-16,1.72,3.6));
#8592=CARTESIAN_POINT('Origin',(1.11022302462516E-16,1.72,2.9));
#8593=CARTESIAN_POINT('Origin',(1.72,0.,2.9));
#8594=CARTESIAN_POINT('',(1.555,-2.02066721859313E-17,2.9));
#8595=CARTESIAN_POINT('Origin',(1.72,0.,2.9));
#8596=CARTESIAN_POINT('',(1.555,2.02066721859313E-17,3.6));
#8597=CARTESIAN_POINT('',(1.555,-2.02066721859313E-17,2.9));
#8598=CARTESIAN_POINT('Origin',(1.72,0.,3.6));
#8599=CARTESIAN_POINT('Origin',(1.72,0.,2.9));
#8600=CARTESIAN_POINT('Origin',(-3.15958874180017E-16,-1.72,2.9));
#8601=CARTESIAN_POINT('',(-0.165,-1.72,2.9));
#8602=CARTESIAN_POINT('Origin',(-3.15958874180017E-16,-1.72,2.9));
#8603=CARTESIAN_POINT('',(-0.165,-1.72,3.6));
#8604=CARTESIAN_POINT('',(-0.165,-1.72,2.9));
#8605=CARTESIAN_POINT('Origin',(-3.15958874180017E-16,-1.72,3.6));
#8606=CARTESIAN_POINT('Origin',(-3.05311331771918E-16,-1.72,2.9));
#8607=CARTESIAN_POINT('Origin',(0.,0.,2.05));
#8608=CARTESIAN_POINT('',(-1.5,-1.83697019872103E-16,2.05));
#8609=CARTESIAN_POINT('Origin',(0.,0.,2.05));
#8610=CARTESIAN_POINT('',(-1.5,1.83697019872103E-16,3.6));
#8611=CARTESIAN_POINT('',(-1.5,-1.83697019872103E-16,2.05));
#8612=CARTESIAN_POINT('Origin',(0.,0.,3.6));
#8613=CARTESIAN_POINT('Origin',(0.,0.,2.05));
#8614=CARTESIAN_POINT('',(-1.02,-1.2491397351303E-16,2.05));
#8615=CARTESIAN_POINT('Origin',(0.,0.,2.05));
#8616=CARTESIAN_POINT('Origin',(0.,0.,0.9));
#8617=CARTESIAN_POINT('',(-1.02,-1.2491397351303E-16,1.));
#8618=CARTESIAN_POINT('Origin',(0.,0.,1.));
#8619=CARTESIAN_POINT('',(-1.02,-1.2491397351303E-16,0.9));
#8620=CARTESIAN_POINT('',(-0.25,-0.988888264668967,1.4));
#8621=CARTESIAN_POINT('Ctrl Pts',(-0.25,-0.988888264668967,1.4));
#8622=CARTESIAN_POINT('Ctrl Pts',(-0.25,-0.988888264668967,1.36846860584118));
#8623=CARTESIAN_POINT('Ctrl Pts',(-0.243672048431404,-0.990553370646674,
1.33492785033683));
#8624=CARTESIAN_POINT('Ctrl Pts',(-0.218119830014375,-0.996491737296663,
1.27337379025046));
#8625=CARTESIAN_POINT('Ctrl Pts',(-0.198902128206072,-1.00067109353237,
1.2453487376128));
#8626=CARTESIAN_POINT('Ctrl Pts',(-0.154654113568716,-1.00845756932386,
1.20110072297544));
#8627=CARTESIAN_POINT('Ctrl Pts',(-0.126627870945253,-1.01258144235289,
1.18188079690607));
#8628=CARTESIAN_POINT('Ctrl Pts',(-0.0650696003913631,-1.0183917429657,
1.15632695599232));
#8629=CARTESIAN_POINT('Ctrl Pts',(-0.031527330883376,-1.02,1.15));
#8630=CARTESIAN_POINT('Ctrl Pts',(0.031527330883376,-1.02,1.15));
#8631=CARTESIAN_POINT('Ctrl Pts',(0.065069600391363,-1.0183917429657,1.15632695599232));
#8632=CARTESIAN_POINT('Ctrl Pts',(0.126627870945253,-1.01258144235289,1.18188079690607));
#8633=CARTESIAN_POINT('Ctrl Pts',(0.154654113568716,-1.00845756932386,1.20110072297544));
#8634=CARTESIAN_POINT('Ctrl Pts',(0.198902128206072,-1.00067109353237,1.2453487376128));
#8635=CARTESIAN_POINT('Ctrl Pts',(0.218119830014375,-0.996491737296663,
1.27337379025046));
#8636=CARTESIAN_POINT('Ctrl Pts',(0.243672048431404,-0.990553370646674,
1.33492785033683));
#8637=CARTESIAN_POINT('Ctrl Pts',(0.25,-0.988888264668967,1.36846860584118));
#8638=CARTESIAN_POINT('Ctrl Pts',(0.25,-0.988888264668967,1.43153139415882));
#8639=CARTESIAN_POINT('Ctrl Pts',(0.243672048431404,-0.990553370646674,
1.46507214966317));
#8640=CARTESIAN_POINT('Ctrl Pts',(0.218119830014375,-0.996491737296663,
1.52662620974954));
#8641=CARTESIAN_POINT('Ctrl Pts',(0.198902128206072,-1.00067109353237,1.5546512623872));
#8642=CARTESIAN_POINT('Ctrl Pts',(0.154654113568716,-1.00845756932386,1.59889927702456));
#8643=CARTESIAN_POINT('Ctrl Pts',(0.126627870945253,-1.01258144235289,1.61811920309393));
#8644=CARTESIAN_POINT('Ctrl Pts',(0.065069600391363,-1.0183917429657,1.64367304400768));
#8645=CARTESIAN_POINT('Ctrl Pts',(0.031527330883376,-1.02,1.65));
#8646=CARTESIAN_POINT('Ctrl Pts',(-0.031527330883376,-1.02,1.65));
#8647=CARTESIAN_POINT('Ctrl Pts',(-0.065069600391363,-1.0183917429657,1.64367304400768));
#8648=CARTESIAN_POINT('Ctrl Pts',(-0.126627870945253,-1.01258144235289,
1.61811920309393));
#8649=CARTESIAN_POINT('Ctrl Pts',(-0.154654113568716,-1.00845756932386,
1.59889927702456));
#8650=CARTESIAN_POINT('Ctrl Pts',(-0.198902128206072,-1.00067109353237,
1.5546512623872));
#8651=CARTESIAN_POINT('Ctrl Pts',(-0.218119830014375,-0.996491737296663,
1.52662620974954));
#8652=CARTESIAN_POINT('Ctrl Pts',(-0.243672048431404,-0.990553370646674,
1.46507214966317));
#8653=CARTESIAN_POINT('Ctrl Pts',(-0.25,-0.988888264668966,1.43153139415882));
#8654=CARTESIAN_POINT('Ctrl Pts',(-0.25,-0.988888264668966,1.4));
#8655=CARTESIAN_POINT('Origin',(5.94264068711928,-1.7,2.2));
#8656=CARTESIAN_POINT('',(5.44264068711928,-1.7,2.2));
#8657=CARTESIAN_POINT('Origin',(5.94264068711928,-1.7,2.2));
#8658=CARTESIAN_POINT('',(5.44264068711928,-1.7,3.6));
#8659=CARTESIAN_POINT('',(5.44264068711928,-1.7,2.2));
#8660=CARTESIAN_POINT('Origin',(5.94264068711928,-1.7,3.6));
#8661=CARTESIAN_POINT('Origin',(5.94264068711928,-1.7,2.2));
#8662=CARTESIAN_POINT('',(5.66764068711928,-1.7,2.2));
#8663=CARTESIAN_POINT('Origin',(5.94264068711928,-1.7,2.2));
#8664=CARTESIAN_POINT('Origin',(-1.7,1.7,2.2));
#8665=CARTESIAN_POINT('',(-2.2,1.7,2.2));
#8666=CARTESIAN_POINT('Origin',(-1.7,1.7,2.2));
#8667=CARTESIAN_POINT('',(-2.2,1.7,3.6));
#8668=CARTESIAN_POINT('',(-2.2,1.7,2.2));
#8669=CARTESIAN_POINT('Origin',(-1.7,1.7,3.6));
#8670=CARTESIAN_POINT('Origin',(-1.7,1.7,2.2));
#8671=CARTESIAN_POINT('',(-1.975,1.7,2.2));
#8672=CARTESIAN_POINT('Origin',(-1.7,1.7,2.2));
#8673=CARTESIAN_POINT('Origin',(-1.7,-1.7,2.2));
#8674=CARTESIAN_POINT('',(-2.2,-1.7,2.2));
#8675=CARTESIAN_POINT('Origin',(-1.7,-1.7,2.2));
#8676=CARTESIAN_POINT('',(-2.2,-1.7,3.6));
#8677=CARTESIAN_POINT('',(-2.2,-1.7,2.2));
#8678=CARTESIAN_POINT('Origin',(-1.7,-1.7,3.6));
#8679=CARTESIAN_POINT('Origin',(-1.7,-1.7,2.2));
#8680=CARTESIAN_POINT('',(-1.975,-1.7,2.2));
#8681=CARTESIAN_POINT('Origin',(-1.7,-1.7,2.2));
#8682=CARTESIAN_POINT('Origin',(5.94264068711928,1.7,2.2));
#8683=CARTESIAN_POINT('',(5.44264068711928,1.7,2.2));
#8684=CARTESIAN_POINT('Origin',(5.94264068711928,1.7,2.2));
#8685=CARTESIAN_POINT('',(5.44264068711928,1.7,3.6));
#8686=CARTESIAN_POINT('',(5.44264068711928,1.7,2.2));
#8687=CARTESIAN_POINT('Origin',(5.94264068711928,1.7,3.6));
#8688=CARTESIAN_POINT('Origin',(5.94264068711928,1.7,2.2));
#8689=CARTESIAN_POINT('',(5.66764068711928,1.7,2.2));
#8690=CARTESIAN_POINT('Origin',(5.94264068711928,1.7,2.2));
#8691=CARTESIAN_POINT('Origin',(5.94264068711928,-1.7,0.9));
#8692=CARTESIAN_POINT('',(5.66764068711928,-1.7,1.));
#8693=CARTESIAN_POINT('Origin',(5.94264068711928,-1.7,1.));
#8694=CARTESIAN_POINT('',(5.66764068711928,-1.7,0.9));
#8695=CARTESIAN_POINT('Origin',(-1.7,1.7,0.9));
#8696=CARTESIAN_POINT('',(-1.975,1.7,1.));
#8697=CARTESIAN_POINT('Origin',(-1.7,1.7,1.));
#8698=CARTESIAN_POINT('',(-1.975,1.7,0.9));
#8699=CARTESIAN_POINT('Origin',(-1.7,-1.7,0.9));
#8700=CARTESIAN_POINT('',(-1.975,-1.7,1.));
#8701=CARTESIAN_POINT('Origin',(-1.7,-1.7,1.));
#8702=CARTESIAN_POINT('',(-1.975,-1.7,0.9));
#8703=CARTESIAN_POINT('Origin',(5.94264068711928,1.7,0.9));
#8704=CARTESIAN_POINT('',(5.66764068711928,1.7,1.));
#8705=CARTESIAN_POINT('Origin',(5.94264068711928,1.7,1.));
#8706=CARTESIAN_POINT('',(5.66764068711928,1.7,0.9));
#8707=CARTESIAN_POINT('Origin',(2.25,0.,1.));
#8708=CARTESIAN_POINT('',(5.73264068711928,1.7,1.));
#8709=CARTESIAN_POINT('Origin',(5.94264068711928,1.7,1.));
#8710=CARTESIAN_POINT('Origin',(2.25,0.,1.));
#8711=CARTESIAN_POINT('',(-1.91,-1.7,1.));
#8712=CARTESIAN_POINT('Origin',(-1.7,-1.7,1.));
#8713=CARTESIAN_POINT('Origin',(2.25,0.,1.));
#8714=CARTESIAN_POINT('',(-1.91,1.7,1.));
#8715=CARTESIAN_POINT('Origin',(-1.7,1.7,1.));
#8716=CARTESIAN_POINT('Origin',(2.25,0.,1.));
#8717=CARTESIAN_POINT('',(5.73264068711928,-1.7,1.));
#8718=CARTESIAN_POINT('Origin',(5.94264068711928,-1.7,1.));
#8719=CARTESIAN_POINT('Origin',(2.25,0.,1.));
#8720=CARTESIAN_POINT('Origin',(2.25,0.,1.));
#8721=CARTESIAN_POINT('Origin',(-2.4,0.,2.3));
#8722=CARTESIAN_POINT('',(-2.4,-2.4,3.6));
#8723=CARTESIAN_POINT('',(-2.4,2.4,3.6));
#8724=CARTESIAN_POINT('',(-2.4,-2.4,3.6));
#8725=CARTESIAN_POINT('',(-2.4,2.4,1.));
#8726=CARTESIAN_POINT('',(-2.4,2.4,3.6));
#8727=CARTESIAN_POINT('',(-2.4,-2.4,1.));
#8728=CARTESIAN_POINT('',(-2.4,0.,1.));
#8729=CARTESIAN_POINT('',(-2.4,-2.4,1.));
#8730=CARTESIAN_POINT('Origin',(2.22132034355964,2.4,2.3));
#8731=CARTESIAN_POINT('',(6.64264068711929,2.4,1.));
#8732=CARTESIAN_POINT('',(0.0249999999999999,2.4,1.));
#8733=CARTESIAN_POINT('',(6.64264068711929,2.4,3.6));
#8734=CARTESIAN_POINT('',(-2.2,2.4,3.6));
#8735=CARTESIAN_POINT('',(6.64264068711929,2.4,3.6));
#8736=CARTESIAN_POINT('Origin',(6.64264068711929,-0.1,2.3));
#8737=CARTESIAN_POINT('',(6.64264068711929,-2.4,1.));
#8738=CARTESIAN_POINT('',(6.64264068711929,1.1,1.));
#8739=CARTESIAN_POINT('',(6.64264068711929,-2.4,3.6));
#8740=CARTESIAN_POINT('',(6.64264068711929,2.2,3.6));
#8741=CARTESIAN_POINT('',(6.64264068711929,-2.4,3.6));
#8742=CARTESIAN_POINT('Origin',(4.24264068711929,-2.2,1.4));
#8743=CARTESIAN_POINT('',(3.99264068711929,-2.4,1.4));
#8744=CARTESIAN_POINT('Origin',(4.24264068711929,-2.4,1.4));
#8745=CARTESIAN_POINT('',(3.99264068711929,-2.2,1.4));
#8746=CARTESIAN_POINT('Origin',(0.,-2.2,1.4));
#8747=CARTESIAN_POINT('',(-0.25,-2.4,1.4));
#8748=CARTESIAN_POINT('Origin',(0.,-2.4,1.4));
#8749=CARTESIAN_POINT('',(-0.25,-2.2,1.4));
#8750=CARTESIAN_POINT('Origin',(6.44264068711929,-2.2,3.6));
#8751=CARTESIAN_POINT('',(6.44264068711928,-2.4,3.6));
#8752=CARTESIAN_POINT('Origin',(2.12132034355964,-2.4,2.3));
#8753=CARTESIAN_POINT('',(0.0249999999999999,-2.4,1.));
#8754=CARTESIAN_POINT('Origin',(9.,-4.3,-0.1));
#8755=CARTESIAN_POINT('',(8.67,-4.3,0.));
#8756=CARTESIAN_POINT('Origin',(9.,-4.3,0.));
#8757=CARTESIAN_POINT('',(8.67,-4.3,1.));
#8758=CARTESIAN_POINT('',(8.67,-4.3,-0.1));
#8759=CARTESIAN_POINT('Origin',(9.,-4.3,1.));
#8760=CARTESIAN_POINT('Origin',(-4.,4.3,-0.1));
#8761=CARTESIAN_POINT('',(-4.33,4.3,0.));
#8762=CARTESIAN_POINT('Origin',(-4.,4.3,0.));
#8763=CARTESIAN_POINT('',(-4.33,4.3,1.));
#8764=CARTESIAN_POINT('',(-4.33,4.3,-0.1));
#8765=CARTESIAN_POINT('Origin',(-4.,4.3,1.));
#8766=CARTESIAN_POINT('Origin',(-4.,-4.3,-0.1));
#8767=CARTESIAN_POINT('',(-4.33,-4.3,0.));
#8768=CARTESIAN_POINT('Origin',(-4.,-4.3,0.));
#8769=CARTESIAN_POINT('',(-4.33,-4.3,1.));
#8770=CARTESIAN_POINT('',(-4.33,-4.3,-0.1));
#8771=CARTESIAN_POINT('Origin',(-4.,-4.3,1.));
#8772=CARTESIAN_POINT('Origin',(9.,4.3,-0.1));
#8773=CARTESIAN_POINT('',(8.67,4.3,0.));
#8774=CARTESIAN_POINT('Origin',(9.,4.3,0.));
#8775=CARTESIAN_POINT('',(8.67,4.3,1.));
#8776=CARTESIAN_POINT('',(8.67,4.3,-0.1));
#8777=CARTESIAN_POINT('Origin',(9.,4.3,1.));
#8778=CARTESIAN_POINT('Origin',(10.,5.,0.));
#8779=CARTESIAN_POINT('',(10.,5.,0.));
#8780=CARTESIAN_POINT('',(-5.,5.,0.));
#8781=CARTESIAN_POINT('',(10.,5.,0.));
#8782=CARTESIAN_POINT('',(-5.,5.,1.));
#8783=CARTESIAN_POINT('',(-5.,5.,0.));
#8784=CARTESIAN_POINT('',(10.,5.,1.));
#8785=CARTESIAN_POINT('',(10.,5.,1.));
#8786=CARTESIAN_POINT('',(10.,5.,0.));
#8787=CARTESIAN_POINT('Origin',(10.,-5.,0.));
#8788=CARTESIAN_POINT('',(10.,-5.,0.));
#8789=CARTESIAN_POINT('',(10.,-5.,0.));
#8790=CARTESIAN_POINT('',(10.,-5.,1.));
#8791=CARTESIAN_POINT('',(10.,-5.,1.));
#8792=CARTESIAN_POINT('',(10.,-5.,0.));
#8793=CARTESIAN_POINT('Origin',(8.,-5.,0.));
#8794=CARTESIAN_POINT('',(-5.,-5.,0.));
#8795=CARTESIAN_POINT('',(-5.,-5.,0.));
#8796=CARTESIAN_POINT('',(-5.,-5.,1.));
#8797=CARTESIAN_POINT('',(-5.,-5.,1.));
#8798=CARTESIAN_POINT('',(-5.,-5.,0.));
#8799=CARTESIAN_POINT('Origin',(-5.,5.,0.));
#8800=CARTESIAN_POINT('',(-5.,5.,0.));
#8801=CARTESIAN_POINT('',(-5.,5.,1.));
#8802=CARTESIAN_POINT('Origin',(5.94264068711928,-1.7,-0.1));
#8803=CARTESIAN_POINT('',(5.73264068711928,-1.7,0.));
#8804=CARTESIAN_POINT('Origin',(5.94264068711928,-1.7,0.));
#8805=CARTESIAN_POINT('',(5.73264068711928,-1.7,-0.1));
#8806=CARTESIAN_POINT('Origin',(-1.7,1.7,-0.1));
#8807=CARTESIAN_POINT('',(-1.91,1.7,0.));
#8808=CARTESIAN_POINT('Origin',(-1.7,1.7,0.));
#8809=CARTESIAN_POINT('',(-1.91,1.7,-0.1));
#8810=CARTESIAN_POINT('Origin',(-1.7,-1.7,-0.1));
#8811=CARTESIAN_POINT('',(-1.91,-1.7,0.));
#8812=CARTESIAN_POINT('Origin',(-1.7,-1.7,0.));
#8813=CARTESIAN_POINT('',(-1.91,-1.7,-0.1));
#8814=CARTESIAN_POINT('Origin',(5.94264068711928,1.7,-0.1));
#8815=CARTESIAN_POINT('',(5.73264068711928,1.7,0.));
#8816=CARTESIAN_POINT('Origin',(5.94264068711928,1.7,0.));
#8817=CARTESIAN_POINT('',(5.73264068711928,1.7,-0.1));
#8818=CARTESIAN_POINT('Origin',(2.25,0.,1.));
#8819=CARTESIAN_POINT('Origin',(2.25,0.,0.));
#10780=UNCERTAINTY_MEASURE_WITH_UNIT(LENGTH_MEASURE(0.001),#10838,
'DISTANCE_ACCURACY_VALUE',
'Maximum model space distance between geometric entities at asserted c
onnectivities');
#10807=UNCERTAINTY_MEASURE_WITH_UNIT(LENGTH_MEASURE(0.001),#10838,
'DISTANCE_ACCURACY_VALUE',
'Maximum model space distance between geometric entities at asserted c
onnectivities');
#10810=(
GEOMETRIC_REPRESENTATION_CONTEXT(3)
GLOBAL_UNCERTAINTY_ASSIGNED_CONTEXT((#10780))
GLOBAL_UNIT_ASSIGNED_CONTEXT((#10838,#10840,#10841))
REPRESENTATION_CONTEXT('','3D')
);
#10837=(
GEOMETRIC_REPRESENTATION_CONTEXT(3)
GLOBAL_UNCERTAINTY_ASSIGNED_CONTEXT((#10807))
GLOBAL_UNIT_ASSIGNED_CONTEXT((#10838,#10840,#10841))
REPRESENTATION_CONTEXT('','3D')
);
#10838=(
LENGTH_UNIT()
NAMED_UNIT(*)
SI_UNIT(.CENTI.,.METRE.)
);
#10840=(
NAMED_UNIT(*)
PLANE_ANGLE_UNIT()
SI_UNIT($,.RADIAN.)
);
#10841=(
NAMED_UNIT(*)
SI_UNIT($,.STERADIAN.)
SOLID_ANGLE_UNIT()
);
#10844=SHAPE_DEFINITION_REPRESENTATION(#10873,#10943);
#10873=PRODUCT_DEFINITION_SHAPE('',$,#10973);
#10943=SHAPE_REPRESENTATION('',(#5930),#10810);
#10970=PRODUCT_DEFINITION_CONTEXT('part definition',#11059,'design');
#10973=PRODUCT_DEFINITION('Demonstrator base plate',
'Demonstrator base plate',#11002,#10970);
#11002=PRODUCT_DEFINITION_FORMATION('',$,#11063);
#11059=APPLICATION_CONTEXT(
'Core Data for Automotive Mechanical Design Process');
#11060=PRODUCT_CONTEXT('part definition',#11059,'mechanical');
#11063=PRODUCT('Demonstrator base plate','Demonstrator base plate',
'Demonstrator base plate',(#11060));
#11139=COLOUR_RGB('Dark Blue',0.08,0.2,0.34);
#11140=FILL_AREA_STYLE_COLOUR('',#11139);
#11141=FILL_AREA_STYLE('',(#11140));
#11142=SURFACE_STYLE_FILL_AREA(#11141);
#11143=SURFACE_SIDE_STYLE('',(#11142));
#11144=SURFACE_STYLE_USAGE(.BOTH.,#11143);
#11145=PRESENTATION_STYLE_ASSIGNMENT((#11144));
ENDSEC;
END-ISO-10303-21;
